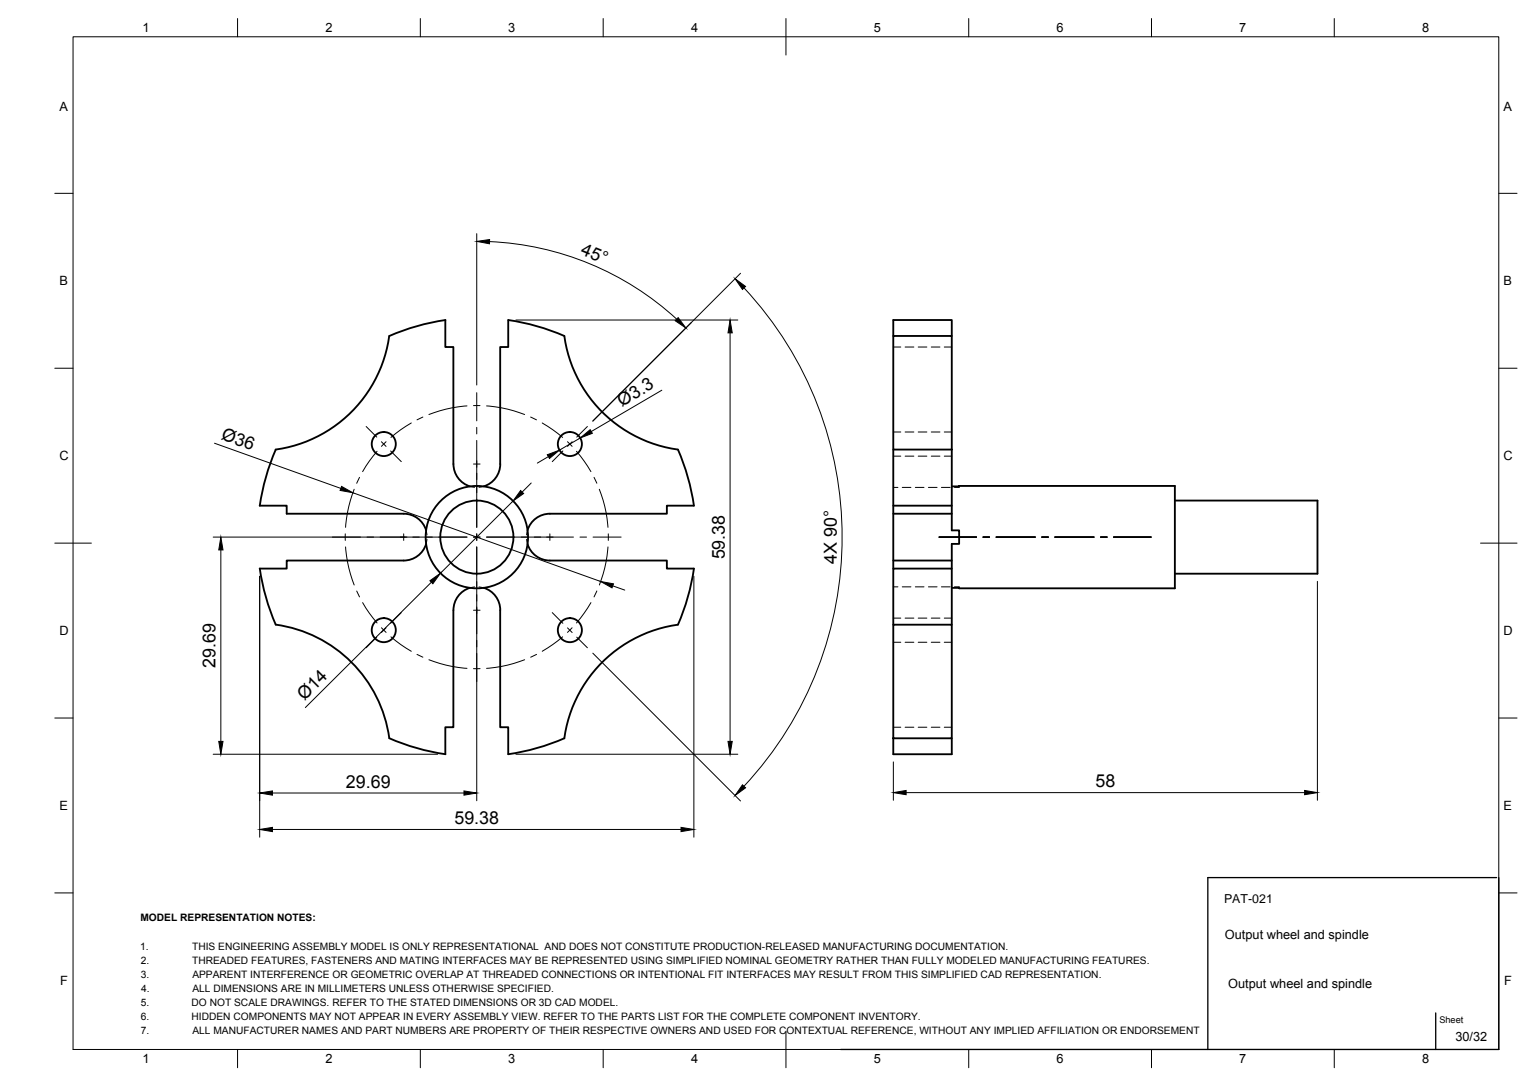
ISO-10303-21;
HEADER;
/* Generated by software containing ST-Developer
 * from STEP Tools, Inc. (www.steptools.com) 
 */

FILE_DESCRIPTION(
/* description */ ('Chain-less indexing wheel (Geneva) drive'),
/* implementation_level */ '2;1');

FILE_NAME(
/* name */ 'Output wheel and spindle.step',
/* time_stamp */ '2026-10-28T03:25:22-07:00',
/* author */ (''),
/* organization */ (''),
/* preprocessor_version */ 'ST-DEVELOPER v20.2',
/* originating_system */ 'Autodesk Translation Framework v15.17.0.0',
/* authorisation */ '');

FILE_SCHEMA (('AUTOMOTIVE_DESIGN { 1 0 10303 214 3 1 1 }'));
ENDSEC;

DATA;
#10=MECHANICAL_DESIGN_GEOMETRIC_PRESENTATION_REPRESENTATION('',(#332),#10957);
#274=SHAPE_REPRESENTATION_RELATIONSHIP('SRR','None',#11090,#299);
#299=ADVANCED_BREP_SHAPE_REPRESENTATION('',(#363),#10953);
#332=STYLED_ITEM('',(#11280),#363);
#363=MANIFOLD_SOLID_BREP('Body1',#5730);
#456=FACE_BOUND('',#1337,.T.);
#457=FACE_BOUND('',#1338,.T.);
#458=FACE_BOUND('',#1339,.T.);
#459=FACE_BOUND('',#1340,.T.);
#460=FACE_BOUND('',#1349,.T.);
#461=FACE_BOUND('',#1351,.T.);
#462=FACE_BOUND('',#1363,.T.);
#463=FACE_BOUND('',#1374,.T.);
#464=FACE_BOUND('',#1388,.T.);
#600=PLANE('',#6604);
#601=PLANE('',#6618);
#602=PLANE('',#6619);
#603=PLANE('',#6620);
#604=PLANE('',#6621);
#605=PLANE('',#6622);
#606=PLANE('',#6623);
#607=PLANE('',#6628);
#608=PLANE('',#6632);
#609=PLANE('',#6644);
#610=PLANE('',#6646);
#611=PLANE('',#6647);
#612=PLANE('',#6648);
#613=PLANE('',#6649);
#614=PLANE('',#6650);
#615=PLANE('',#6651);
#616=PLANE('',#6655);
#617=PLANE('',#6658);
#618=PLANE('',#6660);
#619=PLANE('',#6661);
#620=PLANE('',#6662);
#621=PLANE('',#6663);
#622=PLANE('',#6664);
#623=PLANE('',#6665);
#624=PLANE('',#6669);
#625=PLANE('',#6672);
#626=PLANE('',#6674);
#627=PLANE('',#6675);
#628=PLANE('',#6676);
#629=PLANE('',#6677);
#630=PLANE('',#6678);
#631=PLANE('',#6681);
#632=PLANE('',#6682);
#633=PLANE('',#6683);
#634=PLANE('',#6687);
#903=FACE_OUTER_BOUND('',#1325,.T.);
#904=FACE_OUTER_BOUND('',#1326,.T.);
#905=FACE_OUTER_BOUND('',#1327,.T.);
#906=FACE_OUTER_BOUND('',#1328,.T.);
#907=FACE_OUTER_BOUND('',#1329,.T.);
#908=FACE_OUTER_BOUND('',#1330,.T.);
#909=FACE_OUTER_BOUND('',#1331,.T.);
#910=FACE_OUTER_BOUND('',#1332,.T.);
#911=FACE_OUTER_BOUND('',#1333,.T.);
#912=FACE_OUTER_BOUND('',#1334,.T.);
#913=FACE_OUTER_BOUND('',#1335,.T.);
#914=FACE_OUTER_BOUND('',#1336,.T.);
#915=FACE_OUTER_BOUND('',#1341,.T.);
#916=FACE_OUTER_BOUND('',#1342,.T.);
#917=FACE_OUTER_BOUND('',#1343,.T.);
#918=FACE_OUTER_BOUND('',#1344,.T.);
#919=FACE_OUTER_BOUND('',#1345,.T.);
#920=FACE_OUTER_BOUND('',#1346,.T.);
#921=FACE_OUTER_BOUND('',#1347,.T.);
#922=FACE_OUTER_BOUND('',#1348,.T.);
#923=FACE_OUTER_BOUND('',#1350,.T.);
#924=FACE_OUTER_BOUND('',#1352,.T.);
#925=FACE_OUTER_BOUND('',#1353,.T.);
#926=FACE_OUTER_BOUND('',#1354,.T.);
#927=FACE_OUTER_BOUND('',#1355,.T.);
#928=FACE_OUTER_BOUND('',#1356,.T.);
#929=FACE_OUTER_BOUND('',#1357,.T.);
#930=FACE_OUTER_BOUND('',#1358,.T.);
#931=FACE_OUTER_BOUND('',#1359,.T.);
#932=FACE_OUTER_BOUND('',#1360,.T.);
#933=FACE_OUTER_BOUND('',#1361,.T.);
#934=FACE_OUTER_BOUND('',#1362,.T.);
#935=FACE_OUTER_BOUND('',#1364,.T.);
#936=FACE_OUTER_BOUND('',#1365,.T.);
#937=FACE_OUTER_BOUND('',#1366,.T.);
#938=FACE_OUTER_BOUND('',#1367,.T.);
#939=FACE_OUTER_BOUND('',#1368,.T.);
#940=FACE_OUTER_BOUND('',#1369,.T.);
#941=FACE_OUTER_BOUND('',#1370,.T.);
#942=FACE_OUTER_BOUND('',#1371,.T.);
#943=FACE_OUTER_BOUND('',#1372,.T.);
#944=FACE_OUTER_BOUND('',#1373,.T.);
#945=FACE_OUTER_BOUND('',#1375,.T.);
#946=FACE_OUTER_BOUND('',#1376,.T.);
#947=FACE_OUTER_BOUND('',#1377,.T.);
#948=FACE_OUTER_BOUND('',#1378,.T.);
#949=FACE_OUTER_BOUND('',#1379,.T.);
#950=FACE_OUTER_BOUND('',#1380,.T.);
#951=FACE_OUTER_BOUND('',#1381,.T.);
#952=FACE_OUTER_BOUND('',#1382,.T.);
#953=FACE_OUTER_BOUND('',#1383,.T.);
#954=FACE_OUTER_BOUND('',#1384,.T.);
#955=FACE_OUTER_BOUND('',#1385,.T.);
#956=FACE_OUTER_BOUND('',#1386,.T.);
#957=FACE_OUTER_BOUND('',#1387,.T.);
#958=FACE_OUTER_BOUND('',#1389,.T.);
#959=FACE_OUTER_BOUND('',#1390,.T.);
#1325=EDGE_LOOP('',(#4803,#4804,#4805,#4806));
#1326=EDGE_LOOP('',(#4807,#4808,#4809,#4810));
#1327=EDGE_LOOP('',(#4811,#4812,#4813,#4814));
#1328=EDGE_LOOP('',(#4815,#4816,#4817,#4818));
#1329=EDGE_LOOP('',(#4819,#4820,#4821,#4822));
#1330=EDGE_LOOP('',(#4823,#4824,#4825,#4826));
#1331=EDGE_LOOP('',(#4827,#4828,#4829,#4830));
#1332=EDGE_LOOP('',(#4831,#4832,#4833,#4834));
#1333=EDGE_LOOP('',(#4835,#4836,#4837,#4838));
#1334=EDGE_LOOP('',(#4839,#4840,#4841,#4842));
#1335=EDGE_LOOP('',(#4843,#4844,#4845,#4846));
#1336=EDGE_LOOP('',(#4847,#4848,#4849,#4850,#4851,#4852,#4853,#4854,#4855,
#4856,#4857,#4858,#4859,#4860,#4861,#4862,#4863,#4864,#4865,#4866,#4867,
#4868,#4869,#4870,#4871,#4872,#4873,#4874,#4875,#4876,#4877,#4878,#4879,
#4880,#4881,#4882,#4883,#4884,#4885,#4886));
#1337=EDGE_LOOP('',(#4887));
#1338=EDGE_LOOP('',(#4888));
#1339=EDGE_LOOP('',(#4889));
#1340=EDGE_LOOP('',(#4890));
#1341=EDGE_LOOP('',(#4891,#4892,#4893,#4894));
#1342=EDGE_LOOP('',(#4895,#4896,#4897,#4898));
#1343=EDGE_LOOP('',(#4899,#4900,#4901,#4902));
#1344=EDGE_LOOP('',(#4903,#4904,#4905,#4906));
#1345=EDGE_LOOP('',(#4907,#4908,#4909,#4910));
#1346=EDGE_LOOP('',(#4911,#4912,#4913,#4914));
#1347=EDGE_LOOP('',(#4915,#4916,#4917,#4918));
#1348=EDGE_LOOP('',(#4919,#4920,#4921,#4922,#4923,#4924,#4925,#4926,#4927,
#4928,#4929,#4930));
#1349=EDGE_LOOP('',(#4931));
#1350=EDGE_LOOP('',(#4932,#4933,#4934,#4935,#4936,#4937,#4938,#4939,#4940,
#4941,#4942,#4943));
#1351=EDGE_LOOP('',(#4944));
#1352=EDGE_LOOP('',(#4945,#4946));
#1353=EDGE_LOOP('',(#4947,#4948,#4949,#4950,#4951,#4952,#4953,#4954));
#1354=EDGE_LOOP('',(#4955,#4956,#4957,#4958,#4959,#4960,#4961,#4962,#4963,
#4964,#4965,#4966,#4967,#4968,#4969,#4970,#4971,#4972,#4973,#4974));
#1355=EDGE_LOOP('',(#4975,#4976,#4977,#4978));
#1356=EDGE_LOOP('',(#4979,#4980,#4981,#4982));
#1357=EDGE_LOOP('',(#4983,#4984,#4985,#4986));
#1358=EDGE_LOOP('',(#4987,#4988,#4989,#4990));
#1359=EDGE_LOOP('',(#4991,#4992,#4993,#4994));
#1360=EDGE_LOOP('',(#4995,#4996,#4997,#4998));
#1361=EDGE_LOOP('',(#4999,#5000,#5001,#5002));
#1362=EDGE_LOOP('',(#5003,#5004,#5005,#5006,#5007,#5008,#5009,#5010,#5011,
#5012,#5013,#5014));
#1363=EDGE_LOOP('',(#5015));
#1364=EDGE_LOOP('',(#5016,#5017,#5018));
#1365=EDGE_LOOP('',(#5019,#5020,#5021,#5022,#5023,#5024,#5025,#5026));
#1366=EDGE_LOOP('',(#5027,#5028,#5029,#5030));
#1367=EDGE_LOOP('',(#5031,#5032,#5033,#5034));
#1368=EDGE_LOOP('',(#5035,#5036,#5037,#5038));
#1369=EDGE_LOOP('',(#5039,#5040,#5041,#5042));
#1370=EDGE_LOOP('',(#5043,#5044,#5045,#5046));
#1371=EDGE_LOOP('',(#5047,#5048,#5049,#5050));
#1372=EDGE_LOOP('',(#5051,#5052,#5053,#5054));
#1373=EDGE_LOOP('',(#5055,#5056,#5057,#5058,#5059,#5060,#5061,#5062,#5063,
#5064,#5065,#5066));
#1374=EDGE_LOOP('',(#5067));
#1375=EDGE_LOOP('',(#5068,#5069));
#1376=EDGE_LOOP('',(#5070,#5071,#5072,#5073,#5074,#5075,#5076,#5077));
#1377=EDGE_LOOP('',(#5078,#5079,#5080,#5081));
#1378=EDGE_LOOP('',(#5082,#5083,#5084,#5085));
#1379=EDGE_LOOP('',(#5086,#5087,#5088,#5089));
#1380=EDGE_LOOP('',(#5090,#5091,#5092,#5093));
#1381=EDGE_LOOP('',(#5094,#5095,#5096,#5097));
#1382=EDGE_LOOP('',(#5098,#5099,#5100,#5101));
#1383=EDGE_LOOP('',(#5102,#5103));
#1384=EDGE_LOOP('',(#5104,#5105,#5106,#5107,#5108,#5109,#5110,#5111));
#1385=EDGE_LOOP('',(#5112,#5113,#5114,#5115));
#1386=EDGE_LOOP('',(#5116,#5117,#5118,#5119));
#1387=EDGE_LOOP('',(#5120));
#1388=EDGE_LOOP('',(#5121));
#1389=EDGE_LOOP('',(#5122,#5123,#5124,#5125));
#1390=EDGE_LOOP('',(#5126));
#1663=LINE('',#10310,#2037);
#1664=LINE('',#10316,#2038);
#1665=LINE('',#10322,#2039);
#1666=LINE('',#10328,#2040);
#1667=LINE('',#10335,#2041);
#1668=LINE('',#10338,#2042);
#1669=LINE('',#10344,#2043);
#1670=LINE('',#10347,#2044);
#1671=LINE('',#10353,#2045);
#1672=LINE('',#10356,#2046);
#1673=LINE('',#10360,#2047);
#1674=LINE('',#10364,#2048);
#1675=LINE('',#10370,#2049);
#1676=LINE('',#10376,#2050);
#1677=LINE('',#10382,#2051);
#1678=LINE('',#10386,#2052);
#1679=LINE('',#10388,#2053);
#1680=LINE('',#10390,#2054);
#1681=LINE('',#10394,#2055);
#1682=LINE('',#10396,#2056);
#1683=LINE('',#10398,#2057);
#1684=LINE('',#10403,#2058);
#1685=LINE('',#10405,#2059);
#1686=LINE('',#10407,#2060);
#1687=LINE('',#10411,#2061);
#1688=LINE('',#10413,#2062);
#1689=LINE('',#10415,#2063);
#1690=LINE('',#10418,#2064);
#1691=LINE('',#10420,#2065);
#1692=LINE('',#10422,#2066);
#1693=LINE('',#10426,#2067);
#1694=LINE('',#10428,#2068);
#1695=LINE('',#10430,#2069);
#1696=LINE('',#10433,#2070);
#1697=LINE('',#10435,#2071);
#1698=LINE('',#10437,#2072);
#1699=LINE('',#10441,#2073);
#1700=LINE('',#10443,#2074);
#1701=LINE('',#10445,#2075);
#1702=LINE('',#10450,#2076);
#1703=LINE('',#10453,#2077);
#1704=LINE('',#10457,#2078);
#1705=LINE('',#10458,#2079);
#1706=LINE('',#10461,#2080);
#1707=LINE('',#10462,#2081);
#1708=LINE('',#10465,#2082);
#1709=LINE('',#10467,#2083);
#1710=LINE('',#10468,#2084);
#1711=LINE('',#10470,#2085);
#1712=LINE('',#10473,#2086);
#1713=LINE('',#10474,#2087);
#1714=LINE('',#10479,#2088);
#1715=LINE('',#10481,#2089);
#1716=LINE('',#10483,#2090);
#1717=LINE('',#10491,#2091);
#1718=LINE('',#10499,#2092);
#1719=LINE('',#10501,#2093);
#1720=LINE('',#10502,#2094);
#1721=LINE('',#10509,#2095);
#1722=LINE('',#10510,#2096);
#1723=LINE('',#10511,#2097);
#1724=LINE('',#10514,#2098);
#1725=LINE('',#10518,#2099);
#1726=LINE('',#10523,#2100);
#1727=LINE('',#10527,#2101);
#1728=LINE('',#10531,#2102);
#1729=LINE('',#10535,#2103);
#1730=LINE('',#10538,#2104);
#1731=LINE('',#10541,#2105);
#1732=LINE('',#10543,#2106);
#1733=LINE('',#10545,#2107);
#1734=LINE('',#10548,#2108);
#1735=LINE('',#10550,#2109);
#1736=LINE('',#10551,#2110);
#1737=LINE('',#10553,#2111);
#1738=LINE('',#10556,#2112);
#1739=LINE('',#10557,#2113);
#1740=LINE('',#10562,#2114);
#1741=LINE('',#10564,#2115);
#1742=LINE('',#10566,#2116);
#1743=LINE('',#10572,#2117);
#1744=LINE('',#10575,#2118);
#1745=LINE('',#10577,#2119);
#1746=LINE('',#10579,#2120);
#1747=LINE('',#10582,#2121);
#1748=LINE('',#10584,#2122);
#1749=LINE('',#10585,#2123);
#1750=LINE('',#10587,#2124);
#1751=LINE('',#10590,#2125);
#1752=LINE('',#10591,#2126);
#1753=LINE('',#10596,#2127);
#1754=LINE('',#10598,#2128);
#1755=LINE('',#10600,#2129);
#1756=LINE('',#10606,#2130);
#1757=LINE('',#10609,#2131);
#1758=LINE('',#10611,#2132);
#1759=LINE('',#10613,#2133);
#1760=LINE('',#10615,#2134);
#1761=LINE('',#10617,#2135);
#1762=LINE('',#10621,#2136);
#1763=LINE('',#10622,#2137);
#1764=LINE('',#10630,#2138);
#2037=VECTOR('',#8115,0.165);
#2038=VECTOR('',#8122,0.165);
#2039=VECTOR('',#8129,0.165);
#2040=VECTOR('',#8136,0.165);
#2041=VECTOR('',#8143,1.);
#2042=VECTOR('',#8146,1.);
#2043=VECTOR('',#8151,1.);
#2044=VECTOR('',#8154,1.);
#2045=VECTOR('',#8159,1.);
#2046=VECTOR('',#8162,1.);
#2047=VECTOR('',#8165,1.);
#2048=VECTOR('',#8168,1.);
#2049=VECTOR('',#8175,1.);
#2050=VECTOR('',#8182,1.);
#2051=VECTOR('',#8189,1.);
#2052=VECTOR('',#8194,1.);
#2053=VECTOR('',#8195,1.);
#2054=VECTOR('',#8196,1.);
#2055=VECTOR('',#8199,1.);
#2056=VECTOR('',#8200,1.);
#2057=VECTOR('',#8201,1.);
#2058=VECTOR('',#8206,1.);
#2059=VECTOR('',#8207,1.);
#2060=VECTOR('',#8208,1.);
#2061=VECTOR('',#8211,1.);
#2062=VECTOR('',#8212,1.);
#2063=VECTOR('',#8213,1.);
#2064=VECTOR('',#8216,1.);
#2065=VECTOR('',#8217,1.);
#2066=VECTOR('',#8218,1.);
#2067=VECTOR('',#8221,1.);
#2068=VECTOR('',#8222,1.);
#2069=VECTOR('',#8223,1.);
#2070=VECTOR('',#8226,1.);
#2071=VECTOR('',#8227,1.);
#2072=VECTOR('',#8228,1.);
#2073=VECTOR('',#8231,1.);
#2074=VECTOR('',#8232,1.);
#2075=VECTOR('',#8233,1.);
#2076=VECTOR('',#8240,1.);
#2077=VECTOR('',#8243,1.);
#2078=VECTOR('',#8248,1.);
#2079=VECTOR('',#8249,1.);
#2080=VECTOR('',#8252,1.);
#2081=VECTOR('',#8253,1.);
#2082=VECTOR('',#8256,1.);
#2083=VECTOR('',#8257,1.);
#2084=VECTOR('',#8258,1.);
#2085=VECTOR('',#8261,1.);
#2086=VECTOR('',#8264,1.);
#2087=VECTOR('',#8265,1.);
#2088=VECTOR('',#8270,1.);
#2089=VECTOR('',#8271,1.);
#2090=VECTOR('',#8272,1.);
#2091=VECTOR('',#8281,1.);
#2092=VECTOR('',#8288,1.);
#2093=VECTOR('',#8289,1.);
#2094=VECTOR('',#8290,1.);
#2095=VECTOR('',#8299,1.);
#2096=VECTOR('',#8300,1.);
#2097=VECTOR('',#8301,1.);
#2098=VECTOR('',#8304,1.);
#2099=VECTOR('',#8307,0.7);
#2100=VECTOR('',#8312,1.);
#2101=VECTOR('',#8315,1.);
#2102=VECTOR('',#8318,1.);
#2103=VECTOR('',#8321,1.);
#2104=VECTOR('',#8324,1.);
#2105=VECTOR('',#8329,1.);
#2106=VECTOR('',#8332,1.);
#2107=VECTOR('',#8335,1.);
#2108=VECTOR('',#8338,1.);
#2109=VECTOR('',#8339,1.);
#2110=VECTOR('',#8340,1.);
#2111=VECTOR('',#8343,1.);
#2112=VECTOR('',#8346,1.);
#2113=VECTOR('',#8347,1.);
#2114=VECTOR('',#8352,1.);
#2115=VECTOR('',#8353,1.);
#2116=VECTOR('',#8354,1.);
#2117=VECTOR('',#8365,1.);
#2118=VECTOR('',#8370,1.);
#2119=VECTOR('',#8373,1.);
#2120=VECTOR('',#8376,1.);
#2121=VECTOR('',#8379,1.);
#2122=VECTOR('',#8380,1.);
#2123=VECTOR('',#8381,1.);
#2124=VECTOR('',#8384,1.);
#2125=VECTOR('',#8387,1.);
#2126=VECTOR('',#8388,1.);
#2127=VECTOR('',#8393,1.);
#2128=VECTOR('',#8394,1.);
#2129=VECTOR('',#8395,1.);
#2130=VECTOR('',#8406,1.);
#2131=VECTOR('',#8411,1.);
#2132=VECTOR('',#8414,1.);
#2133=VECTOR('',#8417,1.);
#2134=VECTOR('',#8420,1.);
#2135=VECTOR('',#8423,1.);
#2136=VECTOR('',#8430,1.);
#2137=VECTOR('',#8431,1.);
#2138=VECTOR('',#8442,0.5);
#2429=CIRCLE('',#6572,0.165);
#2430=CIRCLE('',#6573,0.165);
#2431=CIRCLE('',#6575,0.165);
#2432=CIRCLE('',#6576,0.165);
#2433=CIRCLE('',#6578,0.165);
#2434=CIRCLE('',#6579,0.165);
#2435=CIRCLE('',#6581,0.165);
#2436=CIRCLE('',#6582,0.165);
#2437=CIRCLE('',#6584,1.82);
#2438=CIRCLE('',#6585,1.82);
#2439=CIRCLE('',#6587,1.82);
#2440=CIRCLE('',#6588,1.82);
#2441=CIRCLE('',#6590,1.82);
#2442=CIRCLE('',#6591,1.82);
#2443=CIRCLE('',#6593,1.82);
#2444=CIRCLE('',#6594,1.82);
#2445=CIRCLE('',#6596,3.);
#2446=CIRCLE('',#6597,3.);
#2447=CIRCLE('',#6599,3.);
#2448=CIRCLE('',#6600,3.);
#2449=CIRCLE('',#6602,3.);
#2450=CIRCLE('',#6603,3.);
#2451=CIRCLE('',#6605,0.32);
#2452=CIRCLE('',#6606,3.);
#2453=CIRCLE('',#6607,3.);
#2454=CIRCLE('',#6608,0.32);
#2455=CIRCLE('',#6609,3.);
#2456=CIRCLE('',#6610,0.32);
#2457=CIRCLE('',#6611,3.);
#2458=CIRCLE('',#6612,0.32);
#2459=CIRCLE('',#6613,3.);
#2460=CIRCLE('',#6615,3.);
#2461=CIRCLE('',#6617,3.);
#2462=CIRCLE('',#6624,3.);
#2463=CIRCLE('',#6625,0.32);
#2464=CIRCLE('',#6626,0.7);
#2465=CIRCLE('',#6627,0.32);
#2466=CIRCLE('',#6629,0.32);
#2467=CIRCLE('',#6630,0.7);
#2468=CIRCLE('',#6631,0.32);
#2469=CIRCLE('',#6633,0.7);
#2470=CIRCLE('',#6634,0.32);
#2471=CIRCLE('',#6637,0.7);
#2472=CIRCLE('',#6638,0.7);
#2473=CIRCLE('',#6639,0.7);
#2474=CIRCLE('',#6640,0.7);
#2475=CIRCLE('',#6641,0.7);
#2476=CIRCLE('',#6642,0.7);
#2477=CIRCLE('',#6643,0.7);
#2478=CIRCLE('',#6652,3.);
#2479=CIRCLE('',#6653,0.32);
#2480=CIRCLE('',#6654,0.32);
#2481=CIRCLE('',#6656,0.32);
#2482=CIRCLE('',#6666,3.);
#2483=CIRCLE('',#6667,0.32);
#2484=CIRCLE('',#6668,0.32);
#2485=CIRCLE('',#6670,0.32);
#2486=CIRCLE('',#6679,0.32);
#2487=CIRCLE('',#6684,0.5);
#2488=CIRCLE('',#6686,0.5);
#2853=VERTEX_POINT('',#10307);
#2854=VERTEX_POINT('',#10309);
#2855=VERTEX_POINT('',#10313);
#2856=VERTEX_POINT('',#10315);
#2857=VERTEX_POINT('',#10319);
#2858=VERTEX_POINT('',#10321);
#2859=VERTEX_POINT('',#10325);
#2860=VERTEX_POINT('',#10327);
#2861=VERTEX_POINT('',#10331);
#2862=VERTEX_POINT('',#10332);
#2863=VERTEX_POINT('',#10334);
#2864=VERTEX_POINT('',#10336);
#2865=VERTEX_POINT('',#10340);
#2866=VERTEX_POINT('',#10341);
#2867=VERTEX_POINT('',#10343);
#2868=VERTEX_POINT('',#10345);
#2869=VERTEX_POINT('',#10349);
#2870=VERTEX_POINT('',#10350);
#2871=VERTEX_POINT('',#10352);
#2872=VERTEX_POINT('',#10354);
#2873=VERTEX_POINT('',#10358);
#2874=VERTEX_POINT('',#10359);
#2875=VERTEX_POINT('',#10361);
#2876=VERTEX_POINT('',#10363);
#2877=VERTEX_POINT('',#10367);
#2878=VERTEX_POINT('',#10369);
#2879=VERTEX_POINT('',#10373);
#2880=VERTEX_POINT('',#10375);
#2881=VERTEX_POINT('',#10379);
#2882=VERTEX_POINT('',#10381);
#2883=VERTEX_POINT('',#10385);
#2884=VERTEX_POINT('',#10387);
#2885=VERTEX_POINT('',#10389);
#2886=VERTEX_POINT('',#10391);
#2887=VERTEX_POINT('',#10393);
#2888=VERTEX_POINT('',#10395);
#2889=VERTEX_POINT('',#10397);
#2890=VERTEX_POINT('',#10400);
#2891=VERTEX_POINT('',#10402);
#2892=VERTEX_POINT('',#10404);
#2893=VERTEX_POINT('',#10406);
#2894=VERTEX_POINT('',#10408);
#2895=VERTEX_POINT('',#10410);
#2896=VERTEX_POINT('',#10412);
#2897=VERTEX_POINT('',#10414);
#2898=VERTEX_POINT('',#10417);
#2899=VERTEX_POINT('',#10419);
#2900=VERTEX_POINT('',#10421);
#2901=VERTEX_POINT('',#10423);
#2902=VERTEX_POINT('',#10425);
#2903=VERTEX_POINT('',#10427);
#2904=VERTEX_POINT('',#10429);
#2905=VERTEX_POINT('',#10432);
#2906=VERTEX_POINT('',#10434);
#2907=VERTEX_POINT('',#10436);
#2908=VERTEX_POINT('',#10438);
#2909=VERTEX_POINT('',#10440);
#2910=VERTEX_POINT('',#10442);
#2911=VERTEX_POINT('',#10444);
#2912=VERTEX_POINT('',#10448);
#2913=VERTEX_POINT('',#10452);
#2914=VERTEX_POINT('',#10456);
#2915=VERTEX_POINT('',#10460);
#2916=VERTEX_POINT('',#10464);
#2917=VERTEX_POINT('',#10466);
#2918=VERTEX_POINT('',#10472);
#2919=VERTEX_POINT('',#10476);
#2920=VERTEX_POINT('',#10478);
#2921=VERTEX_POINT('',#10480);
#2922=VERTEX_POINT('',#10482);
#2923=VERTEX_POINT('',#10484);
#2924=VERTEX_POINT('',#10486);
#2925=VERTEX_POINT('',#10490);
#2926=VERTEX_POINT('',#10492);
#2927=VERTEX_POINT('',#10494);
#2928=VERTEX_POINT('',#10496);
#2929=VERTEX_POINT('',#10498);
#2930=VERTEX_POINT('',#10500);
#2931=VERTEX_POINT('',#10504);
#2932=VERTEX_POINT('',#10505);
#2933=VERTEX_POINT('',#10513);
#2934=VERTEX_POINT('',#10515);
#2935=VERTEX_POINT('',#10517);
#2936=VERTEX_POINT('',#10520);
#2937=VERTEX_POINT('',#10522);
#2938=VERTEX_POINT('',#10524);
#2939=VERTEX_POINT('',#10526);
#2940=VERTEX_POINT('',#10528);
#2941=VERTEX_POINT('',#10530);
#2942=VERTEX_POINT('',#10532);
#2943=VERTEX_POINT('',#10534);
#2944=VERTEX_POINT('',#10536);
#2945=VERTEX_POINT('',#10547);
#2946=VERTEX_POINT('',#10549);
#2947=VERTEX_POINT('',#10555);
#2948=VERTEX_POINT('',#10559);
#2949=VERTEX_POINT('',#10561);
#2950=VERTEX_POINT('',#10563);
#2951=VERTEX_POINT('',#10565);
#2952=VERTEX_POINT('',#10581);
#2953=VERTEX_POINT('',#10583);
#2954=VERTEX_POINT('',#10589);
#2955=VERTEX_POINT('',#10593);
#2956=VERTEX_POINT('',#10595);
#2957=VERTEX_POINT('',#10597);
#2958=VERTEX_POINT('',#10599);
#2959=VERTEX_POINT('',#10626);
#2960=VERTEX_POINT('',#10629);
#3527=EDGE_CURVE('',#2853,#2853,#2429,.T.);
#3528=EDGE_CURVE('',#2853,#2854,#1663,.T.);
#3529=EDGE_CURVE('',#2854,#2854,#2430,.T.);
#3530=EDGE_CURVE('',#2855,#2855,#2431,.T.);
#3531=EDGE_CURVE('',#2855,#2856,#1664,.T.);
#3532=EDGE_CURVE('',#2856,#2856,#2432,.T.);
#3533=EDGE_CURVE('',#2857,#2857,#2433,.T.);
#3534=EDGE_CURVE('',#2857,#2858,#1665,.T.);
#3535=EDGE_CURVE('',#2858,#2858,#2434,.T.);
#3536=EDGE_CURVE('',#2859,#2859,#2435,.T.);
#3537=EDGE_CURVE('',#2859,#2860,#1666,.T.);
#3538=EDGE_CURVE('',#2860,#2860,#2436,.T.);
#3539=EDGE_CURVE('',#2861,#2862,#2437,.T.);
#3540=EDGE_CURVE('',#2863,#2861,#1667,.T.);
#3541=EDGE_CURVE('',#2864,#2863,#2438,.T.);
#3542=EDGE_CURVE('',#2862,#2864,#1668,.T.);
#3543=EDGE_CURVE('',#2865,#2866,#2439,.T.);
#3544=EDGE_CURVE('',#2867,#2865,#1669,.T.);
#3545=EDGE_CURVE('',#2868,#2867,#2440,.T.);
#3546=EDGE_CURVE('',#2866,#2868,#1670,.T.);
#3547=EDGE_CURVE('',#2869,#2870,#2441,.T.);
#3548=EDGE_CURVE('',#2871,#2869,#1671,.T.);
#3549=EDGE_CURVE('',#2872,#2871,#2442,.T.);
#3550=EDGE_CURVE('',#2870,#2872,#1672,.T.);
#3551=EDGE_CURVE('',#2873,#2874,#1673,.T.);
#3552=EDGE_CURVE('',#2875,#2873,#2443,.T.);
#3553=EDGE_CURVE('',#2876,#2875,#1674,.T.);
#3554=EDGE_CURVE('',#2874,#2876,#2444,.T.);
#3555=EDGE_CURVE('',#2861,#2877,#2445,.T.);
#3556=EDGE_CURVE('',#2877,#2878,#1675,.T.);
#3557=EDGE_CURVE('',#2863,#2878,#2446,.T.);
#3558=EDGE_CURVE('',#2865,#2879,#2447,.T.);
#3559=EDGE_CURVE('',#2879,#2880,#1676,.T.);
#3560=EDGE_CURVE('',#2867,#2880,#2448,.T.);
#3561=EDGE_CURVE('',#2869,#2881,#2449,.T.);
#3562=EDGE_CURVE('',#2881,#2882,#1677,.T.);
#3563=EDGE_CURVE('',#2871,#2882,#2450,.T.);
#3564=EDGE_CURVE('',#2878,#2883,#1678,.T.);
#3565=EDGE_CURVE('',#2883,#2884,#1679,.T.);
#3566=EDGE_CURVE('',#2884,#2885,#1680,.T.);
#3567=EDGE_CURVE('',#2885,#2886,#2451,.T.);
#3568=EDGE_CURVE('',#2886,#2887,#1681,.T.);
#3569=EDGE_CURVE('',#2887,#2888,#1682,.T.);
#3570=EDGE_CURVE('',#2888,#2889,#1683,.T.);
#3571=EDGE_CURVE('',#2889,#2875,#2452,.T.);
#3572=EDGE_CURVE('',#2873,#2890,#2453,.T.);
#3573=EDGE_CURVE('',#2890,#2891,#1684,.T.);
#3574=EDGE_CURVE('',#2891,#2892,#1685,.T.);
#3575=EDGE_CURVE('',#2892,#2893,#1686,.T.);
#3576=EDGE_CURVE('',#2893,#2894,#2454,.T.);
#3577=EDGE_CURVE('',#2894,#2895,#1687,.T.);
#3578=EDGE_CURVE('',#2895,#2896,#1688,.T.);
#3579=EDGE_CURVE('',#2896,#2897,#1689,.T.);
#3580=EDGE_CURVE('',#2897,#2872,#2455,.T.);
#3581=EDGE_CURVE('',#2882,#2898,#1690,.T.);
#3582=EDGE_CURVE('',#2898,#2899,#1691,.T.);
#3583=EDGE_CURVE('',#2899,#2900,#1692,.T.);
#3584=EDGE_CURVE('',#2900,#2901,#2456,.T.);
#3585=EDGE_CURVE('',#2901,#2902,#1693,.T.);
#3586=EDGE_CURVE('',#2902,#2903,#1694,.T.);
#3587=EDGE_CURVE('',#2903,#2904,#1695,.T.);
#3588=EDGE_CURVE('',#2904,#2868,#2457,.T.);
#3589=EDGE_CURVE('',#2880,#2905,#1696,.T.);
#3590=EDGE_CURVE('',#2905,#2906,#1697,.T.);
#3591=EDGE_CURVE('',#2906,#2907,#1698,.T.);
#3592=EDGE_CURVE('',#2907,#2908,#2458,.T.);
#3593=EDGE_CURVE('',#2908,#2909,#1699,.T.);
#3594=EDGE_CURVE('',#2909,#2910,#1700,.T.);
#3595=EDGE_CURVE('',#2910,#2911,#1701,.T.);
#3596=EDGE_CURVE('',#2911,#2864,#2459,.T.);
#3597=EDGE_CURVE('',#2874,#2912,#2460,.T.);
#3598=EDGE_CURVE('',#2912,#2890,#1702,.T.);
#3599=EDGE_CURVE('',#2889,#2913,#1703,.T.);
#3600=EDGE_CURVE('',#2913,#2876,#2461,.T.);
#3601=EDGE_CURVE('',#2914,#2888,#1704,.T.);
#3602=EDGE_CURVE('',#2913,#2914,#1705,.T.);
#3603=EDGE_CURVE('',#2915,#2887,#1706,.T.);
#3604=EDGE_CURVE('',#2914,#2915,#1707,.T.);
#3605=EDGE_CURVE('',#2916,#2883,#1708,.T.);
#3606=EDGE_CURVE('',#2917,#2916,#1709,.T.);
#3607=EDGE_CURVE('',#2884,#2917,#1710,.T.);
#3608=EDGE_CURVE('',#2916,#2877,#1711,.T.);
#3609=EDGE_CURVE('',#2918,#2917,#1712,.T.);
#3610=EDGE_CURVE('',#2918,#2885,#1713,.T.);
#3611=EDGE_CURVE('',#2919,#2862,#2462,.T.);
#3612=EDGE_CURVE('',#2919,#2920,#1714,.T.);
#3613=EDGE_CURVE('',#2920,#2921,#1715,.T.);
#3614=EDGE_CURVE('',#2921,#2922,#1716,.T.);
#3615=EDGE_CURVE('',#2922,#2923,#2463,.T.);
#3616=EDGE_CURVE('',#2923,#2924,#2464,.T.);
#3617=EDGE_CURVE('',#2924,#2918,#2465,.T.);
#3618=EDGE_CURVE('',#2915,#2925,#1717,.T.);
#3619=EDGE_CURVE('',#2925,#2926,#2466,.T.);
#3620=EDGE_CURVE('',#2926,#2927,#2467,.T.);
#3621=EDGE_CURVE('',#2927,#2928,#2468,.T.);
#3622=EDGE_CURVE('',#2928,#2929,#1718,.T.);
#3623=EDGE_CURVE('',#2929,#2930,#1719,.T.);
#3624=EDGE_CURVE('',#2930,#2912,#1720,.T.);
#3625=EDGE_CURVE('',#2931,#2932,#2469,.T.);
#3626=EDGE_CURVE('',#2931,#2932,#2470,.T.);
#3627=EDGE_CURVE('',#2926,#2931,#1721,.T.);
#3628=EDGE_CURVE('',#2925,#2886,#1722,.T.);
#3629=EDGE_CURVE('',#2932,#2924,#1723,.T.);
#3630=EDGE_CURVE('',#2923,#2933,#1724,.T.);
#3631=EDGE_CURVE('',#2933,#2934,#2471,.T.);
#3632=EDGE_CURVE('',#2934,#2935,#1725,.T.);
#3633=EDGE_CURVE('',#2935,#2935,#2472,.T.);
#3634=EDGE_CURVE('',#2934,#2936,#2473,.T.);
#3635=EDGE_CURVE('',#2936,#2937,#1726,.T.);
#3636=EDGE_CURVE('',#2938,#2937,#2474,.T.);
#3637=EDGE_CURVE('',#2938,#2939,#1727,.T.);
#3638=EDGE_CURVE('',#2939,#2940,#2475,.T.);
#3639=EDGE_CURVE('',#2940,#2941,#1728,.T.);
#3640=EDGE_CURVE('',#2942,#2941,#2476,.T.);
#3641=EDGE_CURVE('',#2942,#2943,#1729,.T.);
#3642=EDGE_CURVE('',#2943,#2944,#2477,.T.);
#3643=EDGE_CURVE('',#2944,#2927,#1730,.T.);
#3644=EDGE_CURVE('',#2911,#2919,#1731,.T.);
#3645=EDGE_CURVE('',#2920,#2910,#1732,.T.);
#3646=EDGE_CURVE('',#2921,#2909,#1733,.T.);
#3647=EDGE_CURVE('',#2945,#2905,#1734,.T.);
#3648=EDGE_CURVE('',#2946,#2945,#1735,.T.);
#3649=EDGE_CURVE('',#2906,#2946,#1736,.T.);
#3650=EDGE_CURVE('',#2945,#2879,#1737,.T.);
#3651=EDGE_CURVE('',#2947,#2946,#1738,.T.);
#3652=EDGE_CURVE('',#2947,#2907,#1739,.T.);
#3653=EDGE_CURVE('',#2948,#2866,#2478,.T.);
#3654=EDGE_CURVE('',#2948,#2949,#1740,.T.);
#3655=EDGE_CURVE('',#2949,#2950,#1741,.T.);
#3656=EDGE_CURVE('',#2950,#2951,#1742,.T.);
#3657=EDGE_CURVE('',#2951,#2938,#2479,.T.);
#3658=EDGE_CURVE('',#2937,#2947,#2480,.T.);
#3659=EDGE_CURVE('',#2933,#2936,#2481,.T.);
#3660=EDGE_CURVE('',#2922,#2908,#1743,.T.);
#3661=EDGE_CURVE('',#2904,#2948,#1744,.T.);
#3662=EDGE_CURVE('',#2949,#2903,#1745,.T.);
#3663=EDGE_CURVE('',#2950,#2902,#1746,.T.);
#3664=EDGE_CURVE('',#2952,#2898,#1747,.T.);
#3665=EDGE_CURVE('',#2953,#2952,#1748,.T.);
#3666=EDGE_CURVE('',#2899,#2953,#1749,.T.);
#3667=EDGE_CURVE('',#2952,#2881,#1750,.T.);
#3668=EDGE_CURVE('',#2954,#2953,#1751,.T.);
#3669=EDGE_CURVE('',#2954,#2900,#1752,.T.);
#3670=EDGE_CURVE('',#2955,#2870,#2482,.T.);
#3671=EDGE_CURVE('',#2955,#2956,#1753,.T.);
#3672=EDGE_CURVE('',#2956,#2957,#1754,.T.);
#3673=EDGE_CURVE('',#2957,#2958,#1755,.T.);
#3674=EDGE_CURVE('',#2958,#2942,#2483,.T.);
#3675=EDGE_CURVE('',#2941,#2954,#2484,.T.);
#3676=EDGE_CURVE('',#2939,#2940,#2485,.T.);
#3677=EDGE_CURVE('',#2951,#2901,#1756,.T.);
#3678=EDGE_CURVE('',#2897,#2955,#1757,.T.);
#3679=EDGE_CURVE('',#2956,#2896,#1758,.T.);
#3680=EDGE_CURVE('',#2930,#2891,#1759,.T.);
#3681=EDGE_CURVE('',#2892,#2929,#1760,.T.);
#3682=EDGE_CURVE('',#2957,#2895,#1761,.T.);
#3683=EDGE_CURVE('',#2943,#2944,#2486,.T.);
#3684=EDGE_CURVE('',#2958,#2894,#1762,.T.);
#3685=EDGE_CURVE('',#2928,#2893,#1763,.T.);
#3686=EDGE_CURVE('',#2959,#2959,#2487,.T.);
#3687=EDGE_CURVE('',#2959,#2960,#1764,.T.);
#3688=EDGE_CURVE('',#2960,#2960,#2488,.T.);
#4803=ORIENTED_EDGE('',*,*,#3527,.F.);
#4804=ORIENTED_EDGE('',*,*,#3528,.T.);
#4805=ORIENTED_EDGE('',*,*,#3529,.F.);
#4806=ORIENTED_EDGE('',*,*,#3528,.F.);
#4807=ORIENTED_EDGE('',*,*,#3530,.F.);
#4808=ORIENTED_EDGE('',*,*,#3531,.T.);
#4809=ORIENTED_EDGE('',*,*,#3532,.F.);
#4810=ORIENTED_EDGE('',*,*,#3531,.F.);
#4811=ORIENTED_EDGE('',*,*,#3533,.F.);
#4812=ORIENTED_EDGE('',*,*,#3534,.T.);
#4813=ORIENTED_EDGE('',*,*,#3535,.F.);
#4814=ORIENTED_EDGE('',*,*,#3534,.F.);
#4815=ORIENTED_EDGE('',*,*,#3536,.F.);
#4816=ORIENTED_EDGE('',*,*,#3537,.T.);
#4817=ORIENTED_EDGE('',*,*,#3538,.F.);
#4818=ORIENTED_EDGE('',*,*,#3537,.F.);
#4819=ORIENTED_EDGE('',*,*,#3539,.F.);
#4820=ORIENTED_EDGE('',*,*,#3540,.F.);
#4821=ORIENTED_EDGE('',*,*,#3541,.F.);
#4822=ORIENTED_EDGE('',*,*,#3542,.F.);
#4823=ORIENTED_EDGE('',*,*,#3543,.F.);
#4824=ORIENTED_EDGE('',*,*,#3544,.F.);
#4825=ORIENTED_EDGE('',*,*,#3545,.F.);
#4826=ORIENTED_EDGE('',*,*,#3546,.F.);
#4827=ORIENTED_EDGE('',*,*,#3547,.F.);
#4828=ORIENTED_EDGE('',*,*,#3548,.F.);
#4829=ORIENTED_EDGE('',*,*,#3549,.F.);
#4830=ORIENTED_EDGE('',*,*,#3550,.F.);
#4831=ORIENTED_EDGE('',*,*,#3551,.F.);
#4832=ORIENTED_EDGE('',*,*,#3552,.F.);
#4833=ORIENTED_EDGE('',*,*,#3553,.F.);
#4834=ORIENTED_EDGE('',*,*,#3554,.F.);
#4835=ORIENTED_EDGE('',*,*,#3540,.T.);
#4836=ORIENTED_EDGE('',*,*,#3555,.T.);
#4837=ORIENTED_EDGE('',*,*,#3556,.T.);
#4838=ORIENTED_EDGE('',*,*,#3557,.F.);
#4839=ORIENTED_EDGE('',*,*,#3544,.T.);
#4840=ORIENTED_EDGE('',*,*,#3558,.T.);
#4841=ORIENTED_EDGE('',*,*,#3559,.T.);
#4842=ORIENTED_EDGE('',*,*,#3560,.F.);
#4843=ORIENTED_EDGE('',*,*,#3548,.T.);
#4844=ORIENTED_EDGE('',*,*,#3561,.T.);
#4845=ORIENTED_EDGE('',*,*,#3562,.T.);
#4846=ORIENTED_EDGE('',*,*,#3563,.F.);
#4847=ORIENTED_EDGE('',*,*,#3541,.T.);
#4848=ORIENTED_EDGE('',*,*,#3557,.T.);
#4849=ORIENTED_EDGE('',*,*,#3564,.T.);
#4850=ORIENTED_EDGE('',*,*,#3565,.T.);
#4851=ORIENTED_EDGE('',*,*,#3566,.T.);
#4852=ORIENTED_EDGE('',*,*,#3567,.T.);
#4853=ORIENTED_EDGE('',*,*,#3568,.T.);
#4854=ORIENTED_EDGE('',*,*,#3569,.T.);
#4855=ORIENTED_EDGE('',*,*,#3570,.T.);
#4856=ORIENTED_EDGE('',*,*,#3571,.T.);
#4857=ORIENTED_EDGE('',*,*,#3552,.T.);
#4858=ORIENTED_EDGE('',*,*,#3572,.T.);
#4859=ORIENTED_EDGE('',*,*,#3573,.T.);
#4860=ORIENTED_EDGE('',*,*,#3574,.T.);
#4861=ORIENTED_EDGE('',*,*,#3575,.T.);
#4862=ORIENTED_EDGE('',*,*,#3576,.T.);
#4863=ORIENTED_EDGE('',*,*,#3577,.T.);
#4864=ORIENTED_EDGE('',*,*,#3578,.T.);
#4865=ORIENTED_EDGE('',*,*,#3579,.T.);
#4866=ORIENTED_EDGE('',*,*,#3580,.T.);
#4867=ORIENTED_EDGE('',*,*,#3549,.T.);
#4868=ORIENTED_EDGE('',*,*,#3563,.T.);
#4869=ORIENTED_EDGE('',*,*,#3581,.T.);
#4870=ORIENTED_EDGE('',*,*,#3582,.T.);
#4871=ORIENTED_EDGE('',*,*,#3583,.T.);
#4872=ORIENTED_EDGE('',*,*,#3584,.T.);
#4873=ORIENTED_EDGE('',*,*,#3585,.T.);
#4874=ORIENTED_EDGE('',*,*,#3586,.T.);
#4875=ORIENTED_EDGE('',*,*,#3587,.T.);
#4876=ORIENTED_EDGE('',*,*,#3588,.T.);
#4877=ORIENTED_EDGE('',*,*,#3545,.T.);
#4878=ORIENTED_EDGE('',*,*,#3560,.T.);
#4879=ORIENTED_EDGE('',*,*,#3589,.T.);
#4880=ORIENTED_EDGE('',*,*,#3590,.T.);
#4881=ORIENTED_EDGE('',*,*,#3591,.T.);
#4882=ORIENTED_EDGE('',*,*,#3592,.T.);
#4883=ORIENTED_EDGE('',*,*,#3593,.T.);
#4884=ORIENTED_EDGE('',*,*,#3594,.T.);
#4885=ORIENTED_EDGE('',*,*,#3595,.T.);
#4886=ORIENTED_EDGE('',*,*,#3596,.T.);
#4887=ORIENTED_EDGE('',*,*,#3529,.T.);
#4888=ORIENTED_EDGE('',*,*,#3532,.T.);
#4889=ORIENTED_EDGE('',*,*,#3535,.T.);
#4890=ORIENTED_EDGE('',*,*,#3538,.T.);
#4891=ORIENTED_EDGE('',*,*,#3551,.T.);
#4892=ORIENTED_EDGE('',*,*,#3597,.T.);
#4893=ORIENTED_EDGE('',*,*,#3598,.T.);
#4894=ORIENTED_EDGE('',*,*,#3572,.F.);
#4895=ORIENTED_EDGE('',*,*,#3553,.T.);
#4896=ORIENTED_EDGE('',*,*,#3571,.F.);
#4897=ORIENTED_EDGE('',*,*,#3599,.T.);
#4898=ORIENTED_EDGE('',*,*,#3600,.T.);
#4899=ORIENTED_EDGE('',*,*,#3570,.F.);
#4900=ORIENTED_EDGE('',*,*,#3601,.F.);
#4901=ORIENTED_EDGE('',*,*,#3602,.F.);
#4902=ORIENTED_EDGE('',*,*,#3599,.F.);
#4903=ORIENTED_EDGE('',*,*,#3569,.F.);
#4904=ORIENTED_EDGE('',*,*,#3603,.F.);
#4905=ORIENTED_EDGE('',*,*,#3604,.F.);
#4906=ORIENTED_EDGE('',*,*,#3601,.T.);
#4907=ORIENTED_EDGE('',*,*,#3565,.F.);
#4908=ORIENTED_EDGE('',*,*,#3605,.F.);
#4909=ORIENTED_EDGE('',*,*,#3606,.F.);
#4910=ORIENTED_EDGE('',*,*,#3607,.F.);
#4911=ORIENTED_EDGE('',*,*,#3564,.F.);
#4912=ORIENTED_EDGE('',*,*,#3556,.F.);
#4913=ORIENTED_EDGE('',*,*,#3608,.F.);
#4914=ORIENTED_EDGE('',*,*,#3605,.T.);
#4915=ORIENTED_EDGE('',*,*,#3607,.T.);
#4916=ORIENTED_EDGE('',*,*,#3609,.F.);
#4917=ORIENTED_EDGE('',*,*,#3610,.T.);
#4918=ORIENTED_EDGE('',*,*,#3566,.F.);
#4919=ORIENTED_EDGE('',*,*,#3539,.T.);
#4920=ORIENTED_EDGE('',*,*,#3611,.F.);
#4921=ORIENTED_EDGE('',*,*,#3612,.T.);
#4922=ORIENTED_EDGE('',*,*,#3613,.T.);
#4923=ORIENTED_EDGE('',*,*,#3614,.T.);
#4924=ORIENTED_EDGE('',*,*,#3615,.T.);
#4925=ORIENTED_EDGE('',*,*,#3616,.T.);
#4926=ORIENTED_EDGE('',*,*,#3617,.T.);
#4927=ORIENTED_EDGE('',*,*,#3609,.T.);
#4928=ORIENTED_EDGE('',*,*,#3606,.T.);
#4929=ORIENTED_EDGE('',*,*,#3608,.T.);
#4930=ORIENTED_EDGE('',*,*,#3555,.F.);
#4931=ORIENTED_EDGE('',*,*,#3527,.T.);
#4932=ORIENTED_EDGE('',*,*,#3554,.T.);
#4933=ORIENTED_EDGE('',*,*,#3600,.F.);
#4934=ORIENTED_EDGE('',*,*,#3602,.T.);
#4935=ORIENTED_EDGE('',*,*,#3604,.T.);
#4936=ORIENTED_EDGE('',*,*,#3618,.T.);
#4937=ORIENTED_EDGE('',*,*,#3619,.T.);
#4938=ORIENTED_EDGE('',*,*,#3620,.T.);
#4939=ORIENTED_EDGE('',*,*,#3621,.T.);
#4940=ORIENTED_EDGE('',*,*,#3622,.T.);
#4941=ORIENTED_EDGE('',*,*,#3623,.T.);
#4942=ORIENTED_EDGE('',*,*,#3624,.T.);
#4943=ORIENTED_EDGE('',*,*,#3597,.F.);
#4944=ORIENTED_EDGE('',*,*,#3536,.T.);
#4945=ORIENTED_EDGE('',*,*,#3625,.F.);
#4946=ORIENTED_EDGE('',*,*,#3626,.T.);
#4947=ORIENTED_EDGE('',*,*,#3627,.F.);
#4948=ORIENTED_EDGE('',*,*,#3619,.F.);
#4949=ORIENTED_EDGE('',*,*,#3628,.T.);
#4950=ORIENTED_EDGE('',*,*,#3567,.F.);
#4951=ORIENTED_EDGE('',*,*,#3610,.F.);
#4952=ORIENTED_EDGE('',*,*,#3617,.F.);
#4953=ORIENTED_EDGE('',*,*,#3629,.F.);
#4954=ORIENTED_EDGE('',*,*,#3626,.F.);
#4955=ORIENTED_EDGE('',*,*,#3627,.T.);
#4956=ORIENTED_EDGE('',*,*,#3625,.T.);
#4957=ORIENTED_EDGE('',*,*,#3629,.T.);
#4958=ORIENTED_EDGE('',*,*,#3616,.F.);
#4959=ORIENTED_EDGE('',*,*,#3630,.T.);
#4960=ORIENTED_EDGE('',*,*,#3631,.T.);
#4961=ORIENTED_EDGE('',*,*,#3632,.T.);
#4962=ORIENTED_EDGE('',*,*,#3633,.T.);
#4963=ORIENTED_EDGE('',*,*,#3632,.F.);
#4964=ORIENTED_EDGE('',*,*,#3634,.T.);
#4965=ORIENTED_EDGE('',*,*,#3635,.T.);
#4966=ORIENTED_EDGE('',*,*,#3636,.F.);
#4967=ORIENTED_EDGE('',*,*,#3637,.T.);
#4968=ORIENTED_EDGE('',*,*,#3638,.T.);
#4969=ORIENTED_EDGE('',*,*,#3639,.T.);
#4970=ORIENTED_EDGE('',*,*,#3640,.F.);
#4971=ORIENTED_EDGE('',*,*,#3641,.T.);
#4972=ORIENTED_EDGE('',*,*,#3642,.T.);
#4973=ORIENTED_EDGE('',*,*,#3643,.T.);
#4974=ORIENTED_EDGE('',*,*,#3620,.F.);
#4975=ORIENTED_EDGE('',*,*,#3603,.T.);
#4976=ORIENTED_EDGE('',*,*,#3568,.F.);
#4977=ORIENTED_EDGE('',*,*,#3628,.F.);
#4978=ORIENTED_EDGE('',*,*,#3618,.F.);
#4979=ORIENTED_EDGE('',*,*,#3542,.T.);
#4980=ORIENTED_EDGE('',*,*,#3596,.F.);
#4981=ORIENTED_EDGE('',*,*,#3644,.T.);
#4982=ORIENTED_EDGE('',*,*,#3611,.T.);
#4983=ORIENTED_EDGE('',*,*,#3595,.F.);
#4984=ORIENTED_EDGE('',*,*,#3645,.F.);
#4985=ORIENTED_EDGE('',*,*,#3612,.F.);
#4986=ORIENTED_EDGE('',*,*,#3644,.F.);
#4987=ORIENTED_EDGE('',*,*,#3594,.F.);
#4988=ORIENTED_EDGE('',*,*,#3646,.F.);
#4989=ORIENTED_EDGE('',*,*,#3613,.F.);
#4990=ORIENTED_EDGE('',*,*,#3645,.T.);
#4991=ORIENTED_EDGE('',*,*,#3590,.F.);
#4992=ORIENTED_EDGE('',*,*,#3647,.F.);
#4993=ORIENTED_EDGE('',*,*,#3648,.F.);
#4994=ORIENTED_EDGE('',*,*,#3649,.F.);
#4995=ORIENTED_EDGE('',*,*,#3589,.F.);
#4996=ORIENTED_EDGE('',*,*,#3559,.F.);
#4997=ORIENTED_EDGE('',*,*,#3650,.F.);
#4998=ORIENTED_EDGE('',*,*,#3647,.T.);
#4999=ORIENTED_EDGE('',*,*,#3649,.T.);
#5000=ORIENTED_EDGE('',*,*,#3651,.F.);
#5001=ORIENTED_EDGE('',*,*,#3652,.T.);
#5002=ORIENTED_EDGE('',*,*,#3591,.F.);
#5003=ORIENTED_EDGE('',*,*,#3543,.T.);
#5004=ORIENTED_EDGE('',*,*,#3653,.F.);
#5005=ORIENTED_EDGE('',*,*,#3654,.T.);
#5006=ORIENTED_EDGE('',*,*,#3655,.T.);
#5007=ORIENTED_EDGE('',*,*,#3656,.T.);
#5008=ORIENTED_EDGE('',*,*,#3657,.T.);
#5009=ORIENTED_EDGE('',*,*,#3636,.T.);
#5010=ORIENTED_EDGE('',*,*,#3658,.T.);
#5011=ORIENTED_EDGE('',*,*,#3651,.T.);
#5012=ORIENTED_EDGE('',*,*,#3648,.T.);
#5013=ORIENTED_EDGE('',*,*,#3650,.T.);
#5014=ORIENTED_EDGE('',*,*,#3558,.F.);
#5015=ORIENTED_EDGE('',*,*,#3530,.T.);
#5016=ORIENTED_EDGE('',*,*,#3631,.F.);
#5017=ORIENTED_EDGE('',*,*,#3659,.T.);
#5018=ORIENTED_EDGE('',*,*,#3634,.F.);
#5019=ORIENTED_EDGE('',*,*,#3630,.F.);
#5020=ORIENTED_EDGE('',*,*,#3615,.F.);
#5021=ORIENTED_EDGE('',*,*,#3660,.T.);
#5022=ORIENTED_EDGE('',*,*,#3592,.F.);
#5023=ORIENTED_EDGE('',*,*,#3652,.F.);
#5024=ORIENTED_EDGE('',*,*,#3658,.F.);
#5025=ORIENTED_EDGE('',*,*,#3635,.F.);
#5026=ORIENTED_EDGE('',*,*,#3659,.F.);
#5027=ORIENTED_EDGE('',*,*,#3646,.T.);
#5028=ORIENTED_EDGE('',*,*,#3593,.F.);
#5029=ORIENTED_EDGE('',*,*,#3660,.F.);
#5030=ORIENTED_EDGE('',*,*,#3614,.F.);
#5031=ORIENTED_EDGE('',*,*,#3546,.T.);
#5032=ORIENTED_EDGE('',*,*,#3588,.F.);
#5033=ORIENTED_EDGE('',*,*,#3661,.T.);
#5034=ORIENTED_EDGE('',*,*,#3653,.T.);
#5035=ORIENTED_EDGE('',*,*,#3587,.F.);
#5036=ORIENTED_EDGE('',*,*,#3662,.F.);
#5037=ORIENTED_EDGE('',*,*,#3654,.F.);
#5038=ORIENTED_EDGE('',*,*,#3661,.F.);
#5039=ORIENTED_EDGE('',*,*,#3586,.F.);
#5040=ORIENTED_EDGE('',*,*,#3663,.F.);
#5041=ORIENTED_EDGE('',*,*,#3655,.F.);
#5042=ORIENTED_EDGE('',*,*,#3662,.T.);
#5043=ORIENTED_EDGE('',*,*,#3582,.F.);
#5044=ORIENTED_EDGE('',*,*,#3664,.F.);
#5045=ORIENTED_EDGE('',*,*,#3665,.F.);
#5046=ORIENTED_EDGE('',*,*,#3666,.F.);
#5047=ORIENTED_EDGE('',*,*,#3581,.F.);
#5048=ORIENTED_EDGE('',*,*,#3562,.F.);
#5049=ORIENTED_EDGE('',*,*,#3667,.F.);
#5050=ORIENTED_EDGE('',*,*,#3664,.T.);
#5051=ORIENTED_EDGE('',*,*,#3666,.T.);
#5052=ORIENTED_EDGE('',*,*,#3668,.F.);
#5053=ORIENTED_EDGE('',*,*,#3669,.T.);
#5054=ORIENTED_EDGE('',*,*,#3583,.F.);
#5055=ORIENTED_EDGE('',*,*,#3547,.T.);
#5056=ORIENTED_EDGE('',*,*,#3670,.F.);
#5057=ORIENTED_EDGE('',*,*,#3671,.T.);
#5058=ORIENTED_EDGE('',*,*,#3672,.T.);
#5059=ORIENTED_EDGE('',*,*,#3673,.T.);
#5060=ORIENTED_EDGE('',*,*,#3674,.T.);
#5061=ORIENTED_EDGE('',*,*,#3640,.T.);
#5062=ORIENTED_EDGE('',*,*,#3675,.T.);
#5063=ORIENTED_EDGE('',*,*,#3668,.T.);
#5064=ORIENTED_EDGE('',*,*,#3665,.T.);
#5065=ORIENTED_EDGE('',*,*,#3667,.T.);
#5066=ORIENTED_EDGE('',*,*,#3561,.F.);
#5067=ORIENTED_EDGE('',*,*,#3533,.T.);
#5068=ORIENTED_EDGE('',*,*,#3638,.F.);
#5069=ORIENTED_EDGE('',*,*,#3676,.T.);
#5070=ORIENTED_EDGE('',*,*,#3637,.F.);
#5071=ORIENTED_EDGE('',*,*,#3657,.F.);
#5072=ORIENTED_EDGE('',*,*,#3677,.T.);
#5073=ORIENTED_EDGE('',*,*,#3584,.F.);
#5074=ORIENTED_EDGE('',*,*,#3669,.F.);
#5075=ORIENTED_EDGE('',*,*,#3675,.F.);
#5076=ORIENTED_EDGE('',*,*,#3639,.F.);
#5077=ORIENTED_EDGE('',*,*,#3676,.F.);
#5078=ORIENTED_EDGE('',*,*,#3663,.T.);
#5079=ORIENTED_EDGE('',*,*,#3585,.F.);
#5080=ORIENTED_EDGE('',*,*,#3677,.F.);
#5081=ORIENTED_EDGE('',*,*,#3656,.F.);
#5082=ORIENTED_EDGE('',*,*,#3550,.T.);
#5083=ORIENTED_EDGE('',*,*,#3580,.F.);
#5084=ORIENTED_EDGE('',*,*,#3678,.T.);
#5085=ORIENTED_EDGE('',*,*,#3670,.T.);
#5086=ORIENTED_EDGE('',*,*,#3579,.F.);
#5087=ORIENTED_EDGE('',*,*,#3679,.F.);
#5088=ORIENTED_EDGE('',*,*,#3671,.F.);
#5089=ORIENTED_EDGE('',*,*,#3678,.F.);
#5090=ORIENTED_EDGE('',*,*,#3624,.F.);
#5091=ORIENTED_EDGE('',*,*,#3680,.T.);
#5092=ORIENTED_EDGE('',*,*,#3573,.F.);
#5093=ORIENTED_EDGE('',*,*,#3598,.F.);
#5094=ORIENTED_EDGE('',*,*,#3623,.F.);
#5095=ORIENTED_EDGE('',*,*,#3681,.F.);
#5096=ORIENTED_EDGE('',*,*,#3574,.F.);
#5097=ORIENTED_EDGE('',*,*,#3680,.F.);
#5098=ORIENTED_EDGE('',*,*,#3578,.F.);
#5099=ORIENTED_EDGE('',*,*,#3682,.F.);
#5100=ORIENTED_EDGE('',*,*,#3672,.F.);
#5101=ORIENTED_EDGE('',*,*,#3679,.T.);
#5102=ORIENTED_EDGE('',*,*,#3642,.F.);
#5103=ORIENTED_EDGE('',*,*,#3683,.T.);
#5104=ORIENTED_EDGE('',*,*,#3641,.F.);
#5105=ORIENTED_EDGE('',*,*,#3674,.F.);
#5106=ORIENTED_EDGE('',*,*,#3684,.T.);
#5107=ORIENTED_EDGE('',*,*,#3576,.F.);
#5108=ORIENTED_EDGE('',*,*,#3685,.F.);
#5109=ORIENTED_EDGE('',*,*,#3621,.F.);
#5110=ORIENTED_EDGE('',*,*,#3643,.F.);
#5111=ORIENTED_EDGE('',*,*,#3683,.F.);
#5112=ORIENTED_EDGE('',*,*,#3682,.T.);
#5113=ORIENTED_EDGE('',*,*,#3577,.F.);
#5114=ORIENTED_EDGE('',*,*,#3684,.F.);
#5115=ORIENTED_EDGE('',*,*,#3673,.F.);
#5116=ORIENTED_EDGE('',*,*,#3681,.T.);
#5117=ORIENTED_EDGE('',*,*,#3622,.F.);
#5118=ORIENTED_EDGE('',*,*,#3685,.T.);
#5119=ORIENTED_EDGE('',*,*,#3575,.F.);
#5120=ORIENTED_EDGE('',*,*,#3633,.F.);
#5121=ORIENTED_EDGE('',*,*,#3686,.F.);
#5122=ORIENTED_EDGE('',*,*,#3686,.T.);
#5123=ORIENTED_EDGE('',*,*,#3687,.T.);
#5124=ORIENTED_EDGE('',*,*,#3688,.T.);
#5125=ORIENTED_EDGE('',*,*,#3687,.F.);
#5126=ORIENTED_EDGE('',*,*,#3688,.F.);
#5337=CYLINDRICAL_SURFACE('',#6571,0.165);
#5338=CYLINDRICAL_SURFACE('',#6574,0.165);
#5339=CYLINDRICAL_SURFACE('',#6577,0.165);
#5340=CYLINDRICAL_SURFACE('',#6580,0.165);
#5341=CYLINDRICAL_SURFACE('',#6583,1.82);
#5342=CYLINDRICAL_SURFACE('',#6586,1.82);
#5343=CYLINDRICAL_SURFACE('',#6589,1.82);
#5344=CYLINDRICAL_SURFACE('',#6592,1.82);
#5345=CYLINDRICAL_SURFACE('',#6595,3.);
#5346=CYLINDRICAL_SURFACE('',#6598,3.);
#5347=CYLINDRICAL_SURFACE('',#6601,3.);
#5348=CYLINDRICAL_SURFACE('',#6614,3.);
#5349=CYLINDRICAL_SURFACE('',#6616,3.);
#5350=CYLINDRICAL_SURFACE('',#6635,0.32);
#5351=CYLINDRICAL_SURFACE('',#6636,0.7);
#5352=CYLINDRICAL_SURFACE('',#6645,3.);
#5353=CYLINDRICAL_SURFACE('',#6657,0.32);
#5354=CYLINDRICAL_SURFACE('',#6659,3.);
#5355=CYLINDRICAL_SURFACE('',#6671,0.32);
#5356=CYLINDRICAL_SURFACE('',#6673,3.);
#5357=CYLINDRICAL_SURFACE('',#6680,0.32);
#5358=CYLINDRICAL_SURFACE('',#6685,0.5);
#5617=ADVANCED_FACE('',(#903),#5337,.F.);
#5618=ADVANCED_FACE('',(#904),#5338,.F.);
#5619=ADVANCED_FACE('',(#905),#5339,.F.);
#5620=ADVANCED_FACE('',(#906),#5340,.F.);
#5621=ADVANCED_FACE('',(#907),#5341,.F.);
#5622=ADVANCED_FACE('',(#908),#5342,.F.);
#5623=ADVANCED_FACE('',(#909),#5343,.F.);
#5624=ADVANCED_FACE('',(#910),#5344,.F.);
#5625=ADVANCED_FACE('',(#911),#5345,.T.);
#5626=ADVANCED_FACE('',(#912),#5346,.T.);
#5627=ADVANCED_FACE('',(#913),#5347,.T.);
#5628=ADVANCED_FACE('',(#914,#456,#457,#458,#459),#600,.T.);
#5629=ADVANCED_FACE('',(#915),#5348,.T.);
#5630=ADVANCED_FACE('',(#916),#5349,.T.);
#5631=ADVANCED_FACE('',(#917),#601,.F.);
#5632=ADVANCED_FACE('',(#918),#602,.F.);
#5633=ADVANCED_FACE('',(#919),#603,.F.);
#5634=ADVANCED_FACE('',(#920),#604,.F.);
#5635=ADVANCED_FACE('',(#921),#605,.F.);
#5636=ADVANCED_FACE('',(#922,#460),#606,.F.);
#5637=ADVANCED_FACE('',(#923,#461),#607,.F.);
#5638=ADVANCED_FACE('',(#924),#608,.T.);
#5639=ADVANCED_FACE('',(#925),#5350,.F.);
#5640=ADVANCED_FACE('',(#926),#5351,.T.);
#5641=ADVANCED_FACE('',(#927),#609,.F.);
#5642=ADVANCED_FACE('',(#928),#5352,.T.);
#5643=ADVANCED_FACE('',(#929),#610,.F.);
#5644=ADVANCED_FACE('',(#930),#611,.F.);
#5645=ADVANCED_FACE('',(#931),#612,.F.);
#5646=ADVANCED_FACE('',(#932),#613,.F.);
#5647=ADVANCED_FACE('',(#933),#614,.F.);
#5648=ADVANCED_FACE('',(#934,#462),#615,.F.);
#5649=ADVANCED_FACE('',(#935),#616,.T.);
#5650=ADVANCED_FACE('',(#936),#5353,.F.);
#5651=ADVANCED_FACE('',(#937),#617,.F.);
#5652=ADVANCED_FACE('',(#938),#5354,.T.);
#5653=ADVANCED_FACE('',(#939),#618,.F.);
#5654=ADVANCED_FACE('',(#940),#619,.F.);
#5655=ADVANCED_FACE('',(#941),#620,.F.);
#5656=ADVANCED_FACE('',(#942),#621,.F.);
#5657=ADVANCED_FACE('',(#943),#622,.F.);
#5658=ADVANCED_FACE('',(#944,#463),#623,.F.);
#5659=ADVANCED_FACE('',(#945),#624,.T.);
#5660=ADVANCED_FACE('',(#946),#5355,.F.);
#5661=ADVANCED_FACE('',(#947),#625,.F.);
#5662=ADVANCED_FACE('',(#948),#5356,.T.);
#5663=ADVANCED_FACE('',(#949),#626,.F.);
#5664=ADVANCED_FACE('',(#950),#627,.F.);
#5665=ADVANCED_FACE('',(#951),#628,.F.);
#5666=ADVANCED_FACE('',(#952),#629,.F.);
#5667=ADVANCED_FACE('',(#953),#630,.T.);
#5668=ADVANCED_FACE('',(#954),#5357,.F.);
#5669=ADVANCED_FACE('',(#955),#631,.F.);
#5670=ADVANCED_FACE('',(#956),#632,.F.);
#5671=ADVANCED_FACE('',(#957,#464),#633,.F.);
#5672=ADVANCED_FACE('',(#958),#5358,.T.);
#5673=ADVANCED_FACE('',(#959),#634,.F.);
#5730=CLOSED_SHELL('',(#5617,#5618,#5619,#5620,#5621,#5622,#5623,#5624,
#5625,#5626,#5627,#5628,#5629,#5630,#5631,#5632,#5633,#5634,#5635,#5636,
#5637,#5638,#5639,#5640,#5641,#5642,#5643,#5644,#5645,#5646,#5647,#5648,
#5649,#5650,#5651,#5652,#5653,#5654,#5655,#5656,#5657,#5658,#5659,#5660,
#5661,#5662,#5663,#5664,#5665,#5666,#5667,#5668,#5669,#5670,#5671,#5672,
#5673));
#6570=AXIS2_PLACEMENT_3D('',#10305,#8109,#8110);
#6571=AXIS2_PLACEMENT_3D('',#10306,#8111,#8112);
#6572=AXIS2_PLACEMENT_3D('',#10308,#8113,#8114);
#6573=AXIS2_PLACEMENT_3D('',#10311,#8116,#8117);
#6574=AXIS2_PLACEMENT_3D('',#10312,#8118,#8119);
#6575=AXIS2_PLACEMENT_3D('',#10314,#8120,#8121);
#6576=AXIS2_PLACEMENT_3D('',#10317,#8123,#8124);
#6577=AXIS2_PLACEMENT_3D('',#10318,#8125,#8126);
#6578=AXIS2_PLACEMENT_3D('',#10320,#8127,#8128);
#6579=AXIS2_PLACEMENT_3D('',#10323,#8130,#8131);
#6580=AXIS2_PLACEMENT_3D('',#10324,#8132,#8133);
#6581=AXIS2_PLACEMENT_3D('',#10326,#8134,#8135);
#6582=AXIS2_PLACEMENT_3D('',#10329,#8137,#8138);
#6583=AXIS2_PLACEMENT_3D('',#10330,#8139,#8140);
#6584=AXIS2_PLACEMENT_3D('',#10333,#8141,#8142);
#6585=AXIS2_PLACEMENT_3D('',#10337,#8144,#8145);
#6586=AXIS2_PLACEMENT_3D('',#10339,#8147,#8148);
#6587=AXIS2_PLACEMENT_3D('',#10342,#8149,#8150);
#6588=AXIS2_PLACEMENT_3D('',#10346,#8152,#8153);
#6589=AXIS2_PLACEMENT_3D('',#10348,#8155,#8156);
#6590=AXIS2_PLACEMENT_3D('',#10351,#8157,#8158);
#6591=AXIS2_PLACEMENT_3D('',#10355,#8160,#8161);
#6592=AXIS2_PLACEMENT_3D('',#10357,#8163,#8164);
#6593=AXIS2_PLACEMENT_3D('',#10362,#8166,#8167);
#6594=AXIS2_PLACEMENT_3D('',#10365,#8169,#8170);
#6595=AXIS2_PLACEMENT_3D('',#10366,#8171,#8172);
#6596=AXIS2_PLACEMENT_3D('',#10368,#8173,#8174);
#6597=AXIS2_PLACEMENT_3D('',#10371,#8176,#8177);
#6598=AXIS2_PLACEMENT_3D('',#10372,#8178,#8179);
#6599=AXIS2_PLACEMENT_3D('',#10374,#8180,#8181);
#6600=AXIS2_PLACEMENT_3D('',#10377,#8183,#8184);
#6601=AXIS2_PLACEMENT_3D('',#10378,#8185,#8186);
#6602=AXIS2_PLACEMENT_3D('',#10380,#8187,#8188);
#6603=AXIS2_PLACEMENT_3D('',#10383,#8190,#8191);
#6604=AXIS2_PLACEMENT_3D('',#10384,#8192,#8193);
#6605=AXIS2_PLACEMENT_3D('',#10392,#8197,#8198);
#6606=AXIS2_PLACEMENT_3D('',#10399,#8202,#8203);
#6607=AXIS2_PLACEMENT_3D('',#10401,#8204,#8205);
#6608=AXIS2_PLACEMENT_3D('',#10409,#8209,#8210);
#6609=AXIS2_PLACEMENT_3D('',#10416,#8214,#8215);
#6610=AXIS2_PLACEMENT_3D('',#10424,#8219,#8220);
#6611=AXIS2_PLACEMENT_3D('',#10431,#8224,#8225);
#6612=AXIS2_PLACEMENT_3D('',#10439,#8229,#8230);
#6613=AXIS2_PLACEMENT_3D('',#10446,#8234,#8235);
#6614=AXIS2_PLACEMENT_3D('',#10447,#8236,#8237);
#6615=AXIS2_PLACEMENT_3D('',#10449,#8238,#8239);
#6616=AXIS2_PLACEMENT_3D('',#10451,#8241,#8242);
#6617=AXIS2_PLACEMENT_3D('',#10454,#8244,#8245);
#6618=AXIS2_PLACEMENT_3D('',#10455,#8246,#8247);
#6619=AXIS2_PLACEMENT_3D('',#10459,#8250,#8251);
#6620=AXIS2_PLACEMENT_3D('',#10463,#8254,#8255);
#6621=AXIS2_PLACEMENT_3D('',#10469,#8259,#8260);
#6622=AXIS2_PLACEMENT_3D('',#10471,#8262,#8263);
#6623=AXIS2_PLACEMENT_3D('',#10475,#8266,#8267);
#6624=AXIS2_PLACEMENT_3D('',#10477,#8268,#8269);
#6625=AXIS2_PLACEMENT_3D('',#10485,#8273,#8274);
#6626=AXIS2_PLACEMENT_3D('',#10487,#8275,#8276);
#6627=AXIS2_PLACEMENT_3D('',#10488,#8277,#8278);
#6628=AXIS2_PLACEMENT_3D('',#10489,#8279,#8280);
#6629=AXIS2_PLACEMENT_3D('',#10493,#8282,#8283);
#6630=AXIS2_PLACEMENT_3D('',#10495,#8284,#8285);
#6631=AXIS2_PLACEMENT_3D('',#10497,#8286,#8287);
#6632=AXIS2_PLACEMENT_3D('',#10503,#8291,#8292);
#6633=AXIS2_PLACEMENT_3D('',#10506,#8293,#8294);
#6634=AXIS2_PLACEMENT_3D('',#10507,#8295,#8296);
#6635=AXIS2_PLACEMENT_3D('',#10508,#8297,#8298);
#6636=AXIS2_PLACEMENT_3D('',#10512,#8302,#8303);
#6637=AXIS2_PLACEMENT_3D('',#10516,#8305,#8306);
#6638=AXIS2_PLACEMENT_3D('',#10519,#8308,#8309);
#6639=AXIS2_PLACEMENT_3D('',#10521,#8310,#8311);
#6640=AXIS2_PLACEMENT_3D('',#10525,#8313,#8314);
#6641=AXIS2_PLACEMENT_3D('',#10529,#8316,#8317);
#6642=AXIS2_PLACEMENT_3D('',#10533,#8319,#8320);
#6643=AXIS2_PLACEMENT_3D('',#10537,#8322,#8323);
#6644=AXIS2_PLACEMENT_3D('',#10539,#8325,#8326);
#6645=AXIS2_PLACEMENT_3D('',#10540,#8327,#8328);
#6646=AXIS2_PLACEMENT_3D('',#10542,#8330,#8331);
#6647=AXIS2_PLACEMENT_3D('',#10544,#8333,#8334);
#6648=AXIS2_PLACEMENT_3D('',#10546,#8336,#8337);
#6649=AXIS2_PLACEMENT_3D('',#10552,#8341,#8342);
#6650=AXIS2_PLACEMENT_3D('',#10554,#8344,#8345);
#6651=AXIS2_PLACEMENT_3D('',#10558,#8348,#8349);
#6652=AXIS2_PLACEMENT_3D('',#10560,#8350,#8351);
#6653=AXIS2_PLACEMENT_3D('',#10567,#8355,#8356);
#6654=AXIS2_PLACEMENT_3D('',#10568,#8357,#8358);
#6655=AXIS2_PLACEMENT_3D('',#10569,#8359,#8360);
#6656=AXIS2_PLACEMENT_3D('',#10570,#8361,#8362);
#6657=AXIS2_PLACEMENT_3D('',#10571,#8363,#8364);
#6658=AXIS2_PLACEMENT_3D('',#10573,#8366,#8367);
#6659=AXIS2_PLACEMENT_3D('',#10574,#8368,#8369);
#6660=AXIS2_PLACEMENT_3D('',#10576,#8371,#8372);
#6661=AXIS2_PLACEMENT_3D('',#10578,#8374,#8375);
#6662=AXIS2_PLACEMENT_3D('',#10580,#8377,#8378);
#6663=AXIS2_PLACEMENT_3D('',#10586,#8382,#8383);
#6664=AXIS2_PLACEMENT_3D('',#10588,#8385,#8386);
#6665=AXIS2_PLACEMENT_3D('',#10592,#8389,#8390);
#6666=AXIS2_PLACEMENT_3D('',#10594,#8391,#8392);
#6667=AXIS2_PLACEMENT_3D('',#10601,#8396,#8397);
#6668=AXIS2_PLACEMENT_3D('',#10602,#8398,#8399);
#6669=AXIS2_PLACEMENT_3D('',#10603,#8400,#8401);
#6670=AXIS2_PLACEMENT_3D('',#10604,#8402,#8403);
#6671=AXIS2_PLACEMENT_3D('',#10605,#8404,#8405);
#6672=AXIS2_PLACEMENT_3D('',#10607,#8407,#8408);
#6673=AXIS2_PLACEMENT_3D('',#10608,#8409,#8410);
#6674=AXIS2_PLACEMENT_3D('',#10610,#8412,#8413);
#6675=AXIS2_PLACEMENT_3D('',#10612,#8415,#8416);
#6676=AXIS2_PLACEMENT_3D('',#10614,#8418,#8419);
#6677=AXIS2_PLACEMENT_3D('',#10616,#8421,#8422);
#6678=AXIS2_PLACEMENT_3D('',#10618,#8424,#8425);
#6679=AXIS2_PLACEMENT_3D('',#10619,#8426,#8427);
#6680=AXIS2_PLACEMENT_3D('',#10620,#8428,#8429);
#6681=AXIS2_PLACEMENT_3D('',#10623,#8432,#8433);
#6682=AXIS2_PLACEMENT_3D('',#10624,#8434,#8435);
#6683=AXIS2_PLACEMENT_3D('',#10625,#8436,#8437);
#6684=AXIS2_PLACEMENT_3D('',#10627,#8438,#8439);
#6685=AXIS2_PLACEMENT_3D('',#10628,#8440,#8441);
#6686=AXIS2_PLACEMENT_3D('',#10631,#8443,#8444);
#6687=AXIS2_PLACEMENT_3D('',#10632,#8445,#8446);
#8109=DIRECTION('axis',(0.,0.,1.));
#8110=DIRECTION('refdir',(1.,0.,0.));
#8111=DIRECTION('center_axis',(0.,0.,1.));
#8112=DIRECTION('ref_axis',(1.,0.,0.));
#8113=DIRECTION('center_axis',(0.,0.,1.));
#8114=DIRECTION('ref_axis',(1.,0.,0.));
#8115=DIRECTION('',(0.,0.,1.));
#8116=DIRECTION('center_axis',(0.,0.,-1.));
#8117=DIRECTION('ref_axis',(1.,0.,0.));
#8118=DIRECTION('center_axis',(0.,0.,1.));
#8119=DIRECTION('ref_axis',(1.,0.,0.));
#8120=DIRECTION('center_axis',(0.,0.,1.));
#8121=DIRECTION('ref_axis',(1.,0.,0.));
#8122=DIRECTION('',(0.,0.,1.));
#8123=DIRECTION('center_axis',(0.,0.,-1.));
#8124=DIRECTION('ref_axis',(1.,0.,0.));
#8125=DIRECTION('center_axis',(0.,0.,1.));
#8126=DIRECTION('ref_axis',(1.,0.,0.));
#8127=DIRECTION('center_axis',(0.,0.,1.));
#8128=DIRECTION('ref_axis',(1.,0.,0.));
#8129=DIRECTION('',(0.,0.,1.));
#8130=DIRECTION('center_axis',(0.,0.,-1.));
#8131=DIRECTION('ref_axis',(1.,0.,0.));
#8132=DIRECTION('center_axis',(0.,0.,1.));
#8133=DIRECTION('ref_axis',(1.,0.,0.));
#8134=DIRECTION('center_axis',(0.,0.,1.));
#8135=DIRECTION('ref_axis',(1.,0.,0.));
#8136=DIRECTION('',(0.,0.,1.));
#8137=DIRECTION('center_axis',(0.,0.,-1.));
#8138=DIRECTION('ref_axis',(1.,0.,0.));
#8139=DIRECTION('center_axis',(0.,0.,1.));
#8140=DIRECTION('ref_axis',(1.,0.,0.));
#8141=DIRECTION('center_axis',(0.,0.,1.));
#8142=DIRECTION('ref_axis',(1.,0.,0.));
#8143=DIRECTION('',(0.,0.,-1.));
#8144=DIRECTION('center_axis',(0.,0.,-1.));
#8145=DIRECTION('ref_axis',(1.,0.,0.));
#8146=DIRECTION('',(0.,0.,1.));
#8147=DIRECTION('center_axis',(0.,0.,1.));
#8148=DIRECTION('ref_axis',(1.,0.,0.));
#8149=DIRECTION('center_axis',(0.,0.,1.));
#8150=DIRECTION('ref_axis',(1.,0.,0.));
#8151=DIRECTION('',(0.,0.,-1.));
#8152=DIRECTION('center_axis',(0.,0.,-1.));
#8153=DIRECTION('ref_axis',(1.,0.,0.));
#8154=DIRECTION('',(0.,0.,1.));
#8155=DIRECTION('center_axis',(0.,0.,1.));
#8156=DIRECTION('ref_axis',(1.,0.,0.));
#8157=DIRECTION('center_axis',(0.,0.,1.));
#8158=DIRECTION('ref_axis',(1.,0.,0.));
#8159=DIRECTION('',(0.,0.,-1.));
#8160=DIRECTION('center_axis',(0.,0.,-1.));
#8161=DIRECTION('ref_axis',(1.,0.,0.));
#8162=DIRECTION('',(0.,0.,1.));
#8163=DIRECTION('center_axis',(0.,0.,1.));
#8164=DIRECTION('ref_axis',(1.,0.,0.));
#8165=DIRECTION('',(0.,0.,-1.));
#8166=DIRECTION('center_axis',(0.,0.,-1.));
#8167=DIRECTION('ref_axis',(1.,0.,0.));
#8168=DIRECTION('',(0.,0.,1.));
#8169=DIRECTION('center_axis',(0.,0.,1.));
#8170=DIRECTION('ref_axis',(1.,0.,0.));
#8171=DIRECTION('center_axis',(0.,0.,1.));
#8172=DIRECTION('ref_axis',(1.,0.,0.));
#8173=DIRECTION('center_axis',(0.,0.,1.));
#8174=DIRECTION('ref_axis',(1.,0.,0.));
#8175=DIRECTION('',(0.,0.,1.));
#8176=DIRECTION('center_axis',(0.,0.,1.));
#8177=DIRECTION('ref_axis',(1.,0.,0.));
#8178=DIRECTION('center_axis',(0.,0.,1.));
#8179=DIRECTION('ref_axis',(1.,0.,0.));
#8180=DIRECTION('center_axis',(0.,0.,1.));
#8181=DIRECTION('ref_axis',(1.,0.,0.));
#8182=DIRECTION('',(0.,0.,1.));
#8183=DIRECTION('center_axis',(0.,0.,1.));
#8184=DIRECTION('ref_axis',(1.,0.,0.));
#8185=DIRECTION('center_axis',(0.,0.,1.));
#8186=DIRECTION('ref_axis',(1.,0.,0.));
#8187=DIRECTION('center_axis',(0.,0.,1.));
#8188=DIRECTION('ref_axis',(1.,0.,0.));
#8189=DIRECTION('',(0.,0.,1.));
#8190=DIRECTION('center_axis',(0.,0.,1.));
#8191=DIRECTION('ref_axis',(1.,0.,0.));
#8192=DIRECTION('center_axis',(0.,0.,1.));
#8193=DIRECTION('ref_axis',(1.,0.,0.));
#8194=DIRECTION('',(0.,1.,0.));
#8195=DIRECTION('',(1.,0.,0.));
#8196=DIRECTION('',(1.70803542250024E-16,1.,0.));
#8197=DIRECTION('center_axis',(0.,0.,-1.));
#8198=DIRECTION('ref_axis',(1.,0.,0.));
#8199=DIRECTION('',(-3.41607084500048E-16,-1.,0.));
#8200=DIRECTION('',(1.,0.,0.));
#8201=DIRECTION('',(0.,-1.,0.));
#8202=DIRECTION('center_axis',(0.,0.,1.));
#8203=DIRECTION('ref_axis',(1.,0.,0.));
#8204=DIRECTION('center_axis',(0.,0.,1.));
#8205=DIRECTION('ref_axis',(1.,0.,0.));
#8206=DIRECTION('',(-1.,0.,0.));
#8207=DIRECTION('',(0.,1.,0.));
#8208=DIRECTION('',(-1.,0.,0.));
#8209=DIRECTION('center_axis',(0.,0.,-1.));
#8210=DIRECTION('ref_axis',(1.,0.,0.));
#8211=DIRECTION('',(1.,0.,0.));
#8212=DIRECTION('',(0.,1.,0.));
#8213=DIRECTION('',(1.,0.,0.));
#8214=DIRECTION('center_axis',(0.,0.,1.));
#8215=DIRECTION('ref_axis',(1.,0.,0.));
#8216=DIRECTION('',(0.,-1.,0.));
#8217=DIRECTION('',(-1.,0.,0.));
#8218=DIRECTION('',(0.,-1.,0.));
#8219=DIRECTION('center_axis',(0.,0.,-1.));
#8220=DIRECTION('ref_axis',(1.,0.,0.));
#8221=DIRECTION('',(0.,1.,0.));
#8222=DIRECTION('',(-1.,0.,0.));
#8223=DIRECTION('',(0.,1.,0.));
#8224=DIRECTION('center_axis',(0.,0.,1.));
#8225=DIRECTION('ref_axis',(1.,0.,0.));
#8226=DIRECTION('',(1.,-1.11022302462516E-16,0.));
#8227=DIRECTION('',(0.,-1.,0.));
#8228=DIRECTION('',(1.,-1.06752213906265E-16,0.));
#8229=DIRECTION('center_axis',(0.,0.,-1.));
#8230=DIRECTION('ref_axis',(1.,0.,0.));
#8231=DIRECTION('',(-1.,1.28102656687518E-16,0.));
#8232=DIRECTION('',(0.,-1.,0.));
#8233=DIRECTION('',(-1.,5.55111512312578E-17,0.));
#8234=DIRECTION('center_axis',(0.,0.,1.));
#8235=DIRECTION('ref_axis',(1.,0.,0.));
#8236=DIRECTION('center_axis',(0.,0.,1.));
#8237=DIRECTION('ref_axis',(1.,0.,0.));
#8238=DIRECTION('center_axis',(0.,0.,1.));
#8239=DIRECTION('ref_axis',(1.,0.,0.));
#8240=DIRECTION('',(0.,0.,1.));
#8241=DIRECTION('center_axis',(0.,0.,1.));
#8242=DIRECTION('ref_axis',(1.,0.,0.));
#8243=DIRECTION('',(0.,0.,-1.));
#8244=DIRECTION('center_axis',(0.,0.,1.));
#8245=DIRECTION('ref_axis',(1.,0.,0.));
#8246=DIRECTION('center_axis',(1.,0.,0.));
#8247=DIRECTION('ref_axis',(0.,1.,0.));
#8248=DIRECTION('',(0.,0.,1.));
#8249=DIRECTION('',(0.,1.,0.));
#8250=DIRECTION('center_axis',(0.,1.,0.));
#8251=DIRECTION('ref_axis',(-1.,0.,0.));
#8252=DIRECTION('',(0.,0.,1.));
#8253=DIRECTION('',(-1.,0.,0.));
#8254=DIRECTION('center_axis',(0.,1.,0.));
#8255=DIRECTION('ref_axis',(-1.,0.,0.));
#8256=DIRECTION('',(0.,0.,1.));
#8257=DIRECTION('',(-1.,0.,0.));
#8258=DIRECTION('',(0.,0.,-1.));
#8259=DIRECTION('center_axis',(-1.,0.,0.));
#8260=DIRECTION('ref_axis',(0.,-1.,0.));
#8261=DIRECTION('',(0.,-1.,0.));
#8262=DIRECTION('center_axis',(-1.,1.70803542250024E-16,0.));
#8263=DIRECTION('ref_axis',(-1.70803542250024E-16,-1.,0.));
#8264=DIRECTION('',(-1.70803542250024E-16,-1.,0.));
#8265=DIRECTION('',(0.,0.,1.));
#8266=DIRECTION('center_axis',(0.,0.,1.));
#8267=DIRECTION('ref_axis',(1.,0.,0.));
#8268=DIRECTION('center_axis',(0.,0.,1.));
#8269=DIRECTION('ref_axis',(1.,0.,0.));
#8270=DIRECTION('',(1.,-5.55111512312578E-17,0.));
#8271=DIRECTION('',(0.,1.,0.));
#8272=DIRECTION('',(1.,-1.28102656687518E-16,0.));
#8273=DIRECTION('center_axis',(0.,0.,1.));
#8274=DIRECTION('ref_axis',(1.,0.,0.));
#8275=DIRECTION('center_axis',(0.,0.,1.));
#8276=DIRECTION('ref_axis',(1.,0.,0.));
#8277=DIRECTION('center_axis',(0.,0.,1.));
#8278=DIRECTION('ref_axis',(1.,0.,0.));
#8279=DIRECTION('center_axis',(0.,0.,1.));
#8280=DIRECTION('ref_axis',(1.,0.,0.));
#8281=DIRECTION('',(3.41607084500048E-16,1.,0.));
#8282=DIRECTION('center_axis',(0.,0.,1.));
#8283=DIRECTION('ref_axis',(1.,0.,0.));
#8284=DIRECTION('center_axis',(0.,0.,1.));
#8285=DIRECTION('ref_axis',(1.,0.,0.));
#8286=DIRECTION('center_axis',(0.,0.,1.));
#8287=DIRECTION('ref_axis',(1.,0.,0.));
#8288=DIRECTION('',(1.,0.,0.));
#8289=DIRECTION('',(0.,-1.,0.));
#8290=DIRECTION('',(1.,0.,0.));
#8291=DIRECTION('center_axis',(0.,0.,1.));
#8292=DIRECTION('ref_axis',(1.,0.,0.));
#8293=DIRECTION('center_axis',(0.,0.,-1.));
#8294=DIRECTION('ref_axis',(1.,0.,0.));
#8295=DIRECTION('center_axis',(0.,0.,1.));
#8296=DIRECTION('ref_axis',(1.,0.,0.));
#8297=DIRECTION('center_axis',(0.,0.,1.));
#8298=DIRECTION('ref_axis',(1.,0.,0.));
#8299=DIRECTION('',(0.,0.,-1.));
#8300=DIRECTION('',(0.,0.,1.));
#8301=DIRECTION('',(0.,0.,1.));
#8302=DIRECTION('center_axis',(0.,0.,1.));
#8303=DIRECTION('ref_axis',(1.,0.,0.));
#8304=DIRECTION('',(0.,0.,-1.));
#8305=DIRECTION('center_axis',(0.,0.,-1.));
#8306=DIRECTION('ref_axis',(1.,0.,0.));
#8307=DIRECTION('',(0.,0.,-1.));
#8308=DIRECTION('center_axis',(0.,0.,1.));
#8309=DIRECTION('ref_axis',(1.,0.,0.));
#8310=DIRECTION('center_axis',(0.,0.,-1.));
#8311=DIRECTION('ref_axis',(1.,0.,0.));
#8312=DIRECTION('',(0.,0.,1.));
#8313=DIRECTION('center_axis',(0.,0.,1.));
#8314=DIRECTION('ref_axis',(1.,0.,0.));
#8315=DIRECTION('',(0.,0.,-1.));
#8316=DIRECTION('center_axis',(0.,0.,-1.));
#8317=DIRECTION('ref_axis',(1.,0.,0.));
#8318=DIRECTION('',(0.,0.,1.));
#8319=DIRECTION('center_axis',(0.,0.,1.));
#8320=DIRECTION('ref_axis',(1.,0.,0.));
#8321=DIRECTION('',(0.,0.,-1.));
#8322=DIRECTION('center_axis',(0.,0.,-1.));
#8323=DIRECTION('ref_axis',(1.,0.,0.));
#8324=DIRECTION('',(0.,0.,1.));
#8325=DIRECTION('center_axis',(1.,-3.41607084500048E-16,0.));
#8326=DIRECTION('ref_axis',(3.41607084500048E-16,1.,0.));
#8327=DIRECTION('center_axis',(0.,0.,1.));
#8328=DIRECTION('ref_axis',(1.,0.,0.));
#8329=DIRECTION('',(0.,0.,-1.));
#8330=DIRECTION('center_axis',(-5.55111512312578E-17,-1.,0.));
#8331=DIRECTION('ref_axis',(1.,-5.55111512312578E-17,0.));
#8332=DIRECTION('',(0.,0.,1.));
#8333=DIRECTION('center_axis',(1.,0.,0.));
#8334=DIRECTION('ref_axis',(0.,1.,0.));
#8335=DIRECTION('',(0.,0.,1.));
#8336=DIRECTION('center_axis',(1.,0.,0.));
#8337=DIRECTION('ref_axis',(0.,1.,0.));
#8338=DIRECTION('',(0.,0.,1.));
#8339=DIRECTION('',(0.,1.,0.));
#8340=DIRECTION('',(0.,0.,-1.));
#8341=DIRECTION('center_axis',(1.11022302462516E-16,1.,0.));
#8342=DIRECTION('ref_axis',(-1.,1.11022302462516E-16,0.));
#8343=DIRECTION('',(-1.,1.11022302462516E-16,0.));
#8344=DIRECTION('center_axis',(1.06752213906265E-16,1.,0.));
#8345=DIRECTION('ref_axis',(-1.,1.06752213906265E-16,0.));
#8346=DIRECTION('',(-1.,1.06752213906265E-16,0.));
#8347=DIRECTION('',(0.,0.,1.));
#8348=DIRECTION('center_axis',(0.,0.,1.));
#8349=DIRECTION('ref_axis',(1.,0.,0.));
#8350=DIRECTION('center_axis',(0.,0.,1.));
#8351=DIRECTION('ref_axis',(1.,0.,0.));
#8352=DIRECTION('',(0.,-1.,0.));
#8353=DIRECTION('',(1.,0.,0.));
#8354=DIRECTION('',(0.,-1.,0.));
#8355=DIRECTION('center_axis',(0.,0.,1.));
#8356=DIRECTION('ref_axis',(1.,0.,0.));
#8357=DIRECTION('center_axis',(0.,0.,1.));
#8358=DIRECTION('ref_axis',(1.,0.,0.));
#8359=DIRECTION('center_axis',(0.,0.,1.));
#8360=DIRECTION('ref_axis',(1.,0.,0.));
#8361=DIRECTION('center_axis',(0.,0.,1.));
#8362=DIRECTION('ref_axis',(1.,0.,0.));
#8363=DIRECTION('center_axis',(0.,0.,1.));
#8364=DIRECTION('ref_axis',(1.,0.,0.));
#8365=DIRECTION('',(0.,0.,1.));
#8366=DIRECTION('center_axis',(-1.28102656687518E-16,-1.,0.));
#8367=DIRECTION('ref_axis',(1.,-1.28102656687518E-16,0.));
#8368=DIRECTION('center_axis',(0.,0.,1.));
#8369=DIRECTION('ref_axis',(1.,0.,0.));
#8370=DIRECTION('',(0.,0.,-1.));
#8371=DIRECTION('center_axis',(-1.,0.,0.));
#8372=DIRECTION('ref_axis',(0.,-1.,0.));
#8373=DIRECTION('',(0.,0.,1.));
#8374=DIRECTION('center_axis',(0.,-1.,0.));
#8375=DIRECTION('ref_axis',(1.,0.,0.));
#8376=DIRECTION('',(0.,0.,1.));
#8377=DIRECTION('center_axis',(0.,-1.,0.));
#8378=DIRECTION('ref_axis',(1.,0.,0.));
#8379=DIRECTION('',(0.,0.,1.));
#8380=DIRECTION('',(1.,0.,0.));
#8381=DIRECTION('',(0.,0.,-1.));
#8382=DIRECTION('center_axis',(1.,0.,0.));
#8383=DIRECTION('ref_axis',(0.,1.,0.));
#8384=DIRECTION('',(0.,1.,0.));
#8385=DIRECTION('center_axis',(1.,0.,0.));
#8386=DIRECTION('ref_axis',(0.,1.,0.));
#8387=DIRECTION('',(0.,1.,0.));
#8388=DIRECTION('',(0.,0.,1.));
#8389=DIRECTION('center_axis',(0.,0.,1.));
#8390=DIRECTION('ref_axis',(1.,0.,0.));
#8391=DIRECTION('center_axis',(0.,0.,1.));
#8392=DIRECTION('ref_axis',(1.,0.,0.));
#8393=DIRECTION('',(-1.,0.,0.));
#8394=DIRECTION('',(0.,-1.,0.));
#8395=DIRECTION('',(-1.,0.,0.));
#8396=DIRECTION('center_axis',(0.,0.,1.));
#8397=DIRECTION('ref_axis',(1.,0.,0.));
#8398=DIRECTION('center_axis',(0.,0.,1.));
#8399=DIRECTION('ref_axis',(1.,0.,0.));
#8400=DIRECTION('center_axis',(0.,0.,1.));
#8401=DIRECTION('ref_axis',(1.,0.,0.));
#8402=DIRECTION('center_axis',(0.,0.,1.));
#8403=DIRECTION('ref_axis',(1.,0.,0.));
#8404=DIRECTION('center_axis',(0.,0.,1.));
#8405=DIRECTION('ref_axis',(1.,0.,0.));
#8406=DIRECTION('',(0.,0.,1.));
#8407=DIRECTION('center_axis',(-1.,0.,0.));
#8408=DIRECTION('ref_axis',(0.,-1.,0.));
#8409=DIRECTION('center_axis',(0.,0.,1.));
#8410=DIRECTION('ref_axis',(1.,0.,0.));
#8411=DIRECTION('',(0.,0.,-1.));
#8412=DIRECTION('center_axis',(0.,1.,0.));
#8413=DIRECTION('ref_axis',(-1.,0.,0.));
#8414=DIRECTION('',(0.,0.,1.));
#8415=DIRECTION('center_axis',(0.,-1.,0.));
#8416=DIRECTION('ref_axis',(1.,0.,0.));
#8417=DIRECTION('',(0.,0.,1.));
#8418=DIRECTION('center_axis',(-1.,0.,0.));
#8419=DIRECTION('ref_axis',(0.,-1.,0.));
#8420=DIRECTION('',(0.,0.,-1.));
#8421=DIRECTION('center_axis',(-1.,0.,0.));
#8422=DIRECTION('ref_axis',(0.,-1.,0.));
#8423=DIRECTION('',(0.,0.,1.));
#8424=DIRECTION('center_axis',(0.,0.,1.));
#8425=DIRECTION('ref_axis',(1.,0.,0.));
#8426=DIRECTION('center_axis',(0.,0.,1.));
#8427=DIRECTION('ref_axis',(1.,0.,0.));
#8428=DIRECTION('center_axis',(0.,0.,1.));
#8429=DIRECTION('ref_axis',(-1.,1.22464679914735E-16,0.));
#8430=DIRECTION('',(0.,0.,1.));
#8431=DIRECTION('',(0.,0.,1.));
#8432=DIRECTION('center_axis',(0.,1.,0.));
#8433=DIRECTION('ref_axis',(-1.,0.,0.));
#8434=DIRECTION('center_axis',(0.,-1.,0.));
#8435=DIRECTION('ref_axis',(1.,0.,0.));
#8436=DIRECTION('center_axis',(0.,0.,1.));
#8437=DIRECTION('ref_axis',(1.,0.,0.));
#8438=DIRECTION('center_axis',(0.,0.,-1.));
#8439=DIRECTION('ref_axis',(1.,0.,0.));
#8440=DIRECTION('center_axis',(0.,0.,1.));
#8441=DIRECTION('ref_axis',(1.,0.,0.));
#8442=DIRECTION('',(0.,0.,-1.));
#8443=DIRECTION('center_axis',(0.,0.,1.));
#8444=DIRECTION('ref_axis',(1.,0.,0.));
#8445=DIRECTION('center_axis',(0.,0.,1.));
#8446=DIRECTION('ref_axis',(1.,0.,0.));
#10305=CARTESIAN_POINT('',(0.,0.,0.));
#10306=CARTESIAN_POINT('Origin',(2.9698484809835,-1.27279220613579,5.9));
#10307=CARTESIAN_POINT('',(2.8048484809835,-1.27279220613579,6.));
#10308=CARTESIAN_POINT('Origin',(2.9698484809835,-1.27279220613579,6.));
#10309=CARTESIAN_POINT('',(2.8048484809835,-1.27279220613579,6.8));
#10310=CARTESIAN_POINT('',(2.8048484809835,-1.27279220613579,5.9));
#10311=CARTESIAN_POINT('Origin',(2.9698484809835,-1.27279220613579,6.8));
#10312=CARTESIAN_POINT('Origin',(2.9698484809835,1.27279220613579,5.9));
#10313=CARTESIAN_POINT('',(2.8048484809835,1.27279220613579,6.));
#10314=CARTESIAN_POINT('Origin',(2.9698484809835,1.27279220613579,6.));
#10315=CARTESIAN_POINT('',(2.8048484809835,1.27279220613579,6.8));
#10316=CARTESIAN_POINT('',(2.8048484809835,1.27279220613579,5.9));
#10317=CARTESIAN_POINT('Origin',(2.9698484809835,1.27279220613579,6.8));
#10318=CARTESIAN_POINT('Origin',(5.51543289325507,1.27279220613579,5.9));
#10319=CARTESIAN_POINT('',(5.35043289325507,1.27279220613579,6.));
#10320=CARTESIAN_POINT('Origin',(5.51543289325507,1.27279220613579,6.));
#10321=CARTESIAN_POINT('',(5.35043289325507,1.27279220613579,6.8));
#10322=CARTESIAN_POINT('',(5.35043289325507,1.27279220613579,5.9));
#10323=CARTESIAN_POINT('Origin',(5.51543289325507,1.27279220613579,6.8));
#10324=CARTESIAN_POINT('Origin',(5.51543289325507,-1.27279220613579,5.9));
#10325=CARTESIAN_POINT('',(5.35043289325507,-1.27279220613579,6.));
#10326=CARTESIAN_POINT('Origin',(5.51543289325507,-1.27279220613579,6.));
#10327=CARTESIAN_POINT('',(5.35043289325507,-1.27279220613579,6.8));
#10328=CARTESIAN_POINT('',(5.35043289325507,-1.27279220613579,5.9));
#10329=CARTESIAN_POINT('Origin',(5.51543289325507,-1.27279220613579,6.8));
#10330=CARTESIAN_POINT('Origin',(1.24264068711928,-3.,5.9));
#10331=CARTESIAN_POINT('',(3.04549806673909,-2.75079071295314,6.));
#10332=CARTESIAN_POINT('',(1.49184997416615,-1.19714262038019,6.));
#10333=CARTESIAN_POINT('Origin',(1.24264068711928,-3.,6.));
#10334=CARTESIAN_POINT('',(3.04549806673909,-2.75079071295314,6.8));
#10335=CARTESIAN_POINT('',(3.04549806673909,-2.75079071295314,5.9));
#10336=CARTESIAN_POINT('',(1.49184997416615,-1.19714262038019,6.8));
#10337=CARTESIAN_POINT('Origin',(1.24264068711928,-3.,6.8));
#10338=CARTESIAN_POINT('',(1.49184997416615,-1.19714262038019,5.9));
#10339=CARTESIAN_POINT('Origin',(1.24264068711929,3.,5.9));
#10340=CARTESIAN_POINT('',(1.49184997416615,1.19714262038019,6.));
#10341=CARTESIAN_POINT('',(3.04549806673909,2.75079071295314,6.));
#10342=CARTESIAN_POINT('Origin',(1.24264068711929,3.,6.));
#10343=CARTESIAN_POINT('',(1.49184997416615,1.19714262038019,6.8));
#10344=CARTESIAN_POINT('',(1.49184997416615,1.19714262038019,5.9));
#10345=CARTESIAN_POINT('',(3.04549806673909,2.75079071295314,6.8));
#10346=CARTESIAN_POINT('Origin',(1.24264068711929,3.,6.8));
#10347=CARTESIAN_POINT('',(3.04549806673909,2.75079071295314,5.9));
#10348=CARTESIAN_POINT('Origin',(7.24264068711929,3.,5.9));
#10349=CARTESIAN_POINT('',(5.43978330749948,2.75079071295314,6.));
#10350=CARTESIAN_POINT('',(6.99343140007243,1.19714262038019,6.));
#10351=CARTESIAN_POINT('Origin',(7.24264068711929,3.,6.));
#10352=CARTESIAN_POINT('',(5.43978330749948,2.75079071295314,6.8));
#10353=CARTESIAN_POINT('',(5.43978330749948,2.75079071295314,5.9));
#10354=CARTESIAN_POINT('',(6.99343140007243,1.19714262038019,6.8));
#10355=CARTESIAN_POINT('Origin',(7.24264068711929,3.,6.8));
#10356=CARTESIAN_POINT('',(6.99343140007243,1.19714262038019,5.9));
#10357=CARTESIAN_POINT('Origin',(7.24264068711929,-3.,5.9));
#10358=CARTESIAN_POINT('',(6.99343140007242,-1.19714262038019,6.8));
#10359=CARTESIAN_POINT('',(6.99343140007242,-1.19714262038019,6.));
#10360=CARTESIAN_POINT('',(6.99343140007243,-1.19714262038019,5.9));
#10361=CARTESIAN_POINT('',(5.43978330749948,-2.75079071295314,6.8));
#10362=CARTESIAN_POINT('Origin',(7.24264068711929,-3.,6.8));
#10363=CARTESIAN_POINT('',(5.43978330749948,-2.75079071295314,6.));
#10364=CARTESIAN_POINT('',(5.43978330749948,-2.75079071295314,5.9));
#10365=CARTESIAN_POINT('Origin',(7.24264068711929,-3.,6.));
#10366=CARTESIAN_POINT('Origin',(4.24264068711929,0.,6.));
#10367=CARTESIAN_POINT('',(3.81264068711929,-2.96902340846279,6.));
#10368=CARTESIAN_POINT('Origin',(4.24264068711929,0.,6.));
#10369=CARTESIAN_POINT('',(3.81264068711929,-2.96902340846279,6.8));
#10370=CARTESIAN_POINT('',(3.81264068711929,-2.96902340846279,6.));
#10371=CARTESIAN_POINT('Origin',(4.24264068711929,0.,6.8));
#10372=CARTESIAN_POINT('Origin',(4.24264068711929,0.,6.));
#10373=CARTESIAN_POINT('',(1.2736172786565,0.43,6.));
#10374=CARTESIAN_POINT('Origin',(4.24264068711929,0.,6.));
#10375=CARTESIAN_POINT('',(1.2736172786565,0.43,6.8));
#10376=CARTESIAN_POINT('',(1.2736172786565,0.43,6.));
#10377=CARTESIAN_POINT('Origin',(4.24264068711929,0.,6.8));
#10378=CARTESIAN_POINT('Origin',(4.24264068711929,0.,6.));
#10379=CARTESIAN_POINT('',(4.67264068711929,2.96902340846279,6.));
#10380=CARTESIAN_POINT('Origin',(4.24264068711929,0.,6.));
#10381=CARTESIAN_POINT('',(4.67264068711929,2.96902340846279,6.8));
#10382=CARTESIAN_POINT('',(4.67264068711929,2.96902340846279,6.));
#10383=CARTESIAN_POINT('Origin',(4.24264068711929,0.,6.8));
#10384=CARTESIAN_POINT('Origin',(4.24264068711929,0.,6.8));
#10385=CARTESIAN_POINT('',(3.81264068711929,-2.6,6.8));
#10386=CARTESIAN_POINT('',(3.81264068711929,-1.3,6.8));
#10387=CARTESIAN_POINT('',(3.92264068711928,-2.6,6.8));
#10388=CARTESIAN_POINT('',(4.45764068711929,-2.6,6.8));
#10389=CARTESIAN_POINT('',(3.92264068711928,-1.,6.8));
#10390=CARTESIAN_POINT('',(3.92264068711929,-0.5,6.8));
#10391=CARTESIAN_POINT('',(4.56264068711929,-1.,6.8));
#10392=CARTESIAN_POINT('Origin',(4.24264068711929,-1.,6.8));
#10393=CARTESIAN_POINT('',(4.56264068711929,-2.6,6.8));
#10394=CARTESIAN_POINT('',(4.56264068711929,-1.8,6.8));
#10395=CARTESIAN_POINT('',(4.67264068711928,-2.6,6.8));
#10396=CARTESIAN_POINT('',(4.45764068711929,-2.6,6.8));
#10397=CARTESIAN_POINT('',(4.67264068711928,-2.96902340846279,6.8));
#10398=CARTESIAN_POINT('',(4.67264068711929,-1.8,6.8));
#10399=CARTESIAN_POINT('Origin',(4.24264068711929,0.,6.8));
#10400=CARTESIAN_POINT('',(7.21166409558207,-0.43,6.8));
#10401=CARTESIAN_POINT('Origin',(4.24264068711929,0.,6.8));
#10402=CARTESIAN_POINT('',(6.84264068711929,-0.43,6.8));
#10403=CARTESIAN_POINT('',(5.54264068711929,-0.43,6.8));
#10404=CARTESIAN_POINT('',(6.84264068711929,-0.32,6.8));
#10405=CARTESIAN_POINT('',(6.84264068711929,0.215,6.8));
#10406=CARTESIAN_POINT('',(5.24264068711929,-0.32,6.8));
#10407=CARTESIAN_POINT('',(4.74264068711929,-0.32,6.8));
#10408=CARTESIAN_POINT('',(5.24264068711929,0.32,6.8));
#10409=CARTESIAN_POINT('Origin',(5.24264068711929,0.,6.8));
#10410=CARTESIAN_POINT('',(6.84264068711929,0.32,6.8));
#10411=CARTESIAN_POINT('',(6.04264068711929,0.32,6.8));
#10412=CARTESIAN_POINT('',(6.84264068711929,0.43,6.8));
#10413=CARTESIAN_POINT('',(6.84264068711929,0.215,6.8));
#10414=CARTESIAN_POINT('',(7.21166409558207,0.43,6.8));
#10415=CARTESIAN_POINT('',(6.04264068711929,0.43,6.8));
#10416=CARTESIAN_POINT('Origin',(4.24264068711929,0.,6.8));
#10417=CARTESIAN_POINT('',(4.67264068711929,2.6,6.8));
#10418=CARTESIAN_POINT('',(4.67264068711929,1.3,6.8));
#10419=CARTESIAN_POINT('',(4.56264068711929,2.6,6.8));
#10420=CARTESIAN_POINT('',(4.02764068711929,2.6,6.8));
#10421=CARTESIAN_POINT('',(4.56264068711929,1.,6.8));
#10422=CARTESIAN_POINT('',(4.56264068711929,0.5,6.8));
#10423=CARTESIAN_POINT('',(3.92264068711928,1.,6.8));
#10424=CARTESIAN_POINT('Origin',(4.24264068711929,1.,6.8));
#10425=CARTESIAN_POINT('',(3.92264068711929,2.6,6.8));
#10426=CARTESIAN_POINT('',(3.92264068711929,1.8,6.8));
#10427=CARTESIAN_POINT('',(3.81264068711929,2.6,6.8));
#10428=CARTESIAN_POINT('',(4.02764068711929,2.6,6.8));
#10429=CARTESIAN_POINT('',(3.81264068711929,2.96902340846279,6.8));
#10430=CARTESIAN_POINT('',(3.81264068711929,1.8,6.8));
#10431=CARTESIAN_POINT('Origin',(4.24264068711929,0.,6.8));
#10432=CARTESIAN_POINT('',(1.64264068711929,0.43,6.8));
#10433=CARTESIAN_POINT('',(2.94264068711929,0.43,6.8));
#10434=CARTESIAN_POINT('',(1.64264068711929,0.32,6.8));
#10435=CARTESIAN_POINT('',(1.64264068711929,-0.215,6.8));
#10436=CARTESIAN_POINT('',(3.24264068711929,0.32,6.8));
#10437=CARTESIAN_POINT('',(3.74264068711929,0.32,6.8));
#10438=CARTESIAN_POINT('',(3.24264068711929,-0.32,6.8));
#10439=CARTESIAN_POINT('Origin',(3.24264068711929,1.22464679914735E-16,
6.8));
#10440=CARTESIAN_POINT('',(1.64264068711929,-0.32,6.8));
#10441=CARTESIAN_POINT('',(2.44264068711929,-0.32,6.8));
#10442=CARTESIAN_POINT('',(1.64264068711929,-0.43,6.8));
#10443=CARTESIAN_POINT('',(1.64264068711929,-0.215,6.8));
#10444=CARTESIAN_POINT('',(1.2736172786565,-0.43,6.8));
#10445=CARTESIAN_POINT('',(2.44264068711929,-0.43,6.8));
#10446=CARTESIAN_POINT('Origin',(4.24264068711929,0.,6.8));
#10447=CARTESIAN_POINT('Origin',(4.24264068711929,0.,6.));
#10448=CARTESIAN_POINT('',(7.21166409558207,-0.43,6.));
#10449=CARTESIAN_POINT('Origin',(4.24264068711929,0.,6.));
#10450=CARTESIAN_POINT('',(7.21166409558207,-0.43,6.));
#10451=CARTESIAN_POINT('Origin',(4.24264068711929,0.,6.));
#10452=CARTESIAN_POINT('',(4.67264068711928,-2.96902340846279,6.));
#10453=CARTESIAN_POINT('',(4.67264068711928,-2.96902340846279,6.));
#10454=CARTESIAN_POINT('Origin',(4.24264068711929,0.,6.));
#10455=CARTESIAN_POINT('Origin',(4.67264068711928,-3.6,5.9));
#10456=CARTESIAN_POINT('',(4.67264068711928,-2.6,6.));
#10457=CARTESIAN_POINT('',(4.67264068711928,-2.6,5.9));
#10458=CARTESIAN_POINT('',(4.67264068711929,-1.8,6.));
#10459=CARTESIAN_POINT('Origin',(4.67264068711928,-2.6,5.9));
#10460=CARTESIAN_POINT('',(4.56264068711929,-2.6,6.));
#10461=CARTESIAN_POINT('',(4.56264068711929,-2.6,5.9));
#10462=CARTESIAN_POINT('',(4.45764068711929,-2.6,6.));
#10463=CARTESIAN_POINT('Origin',(4.67264068711928,-2.6,5.9));
#10464=CARTESIAN_POINT('',(3.81264068711929,-2.6,6.));
#10465=CARTESIAN_POINT('',(3.81264068711929,-2.6,5.9));
#10466=CARTESIAN_POINT('',(3.92264068711928,-2.6,6.));
#10467=CARTESIAN_POINT('',(4.45764068711929,-2.6,6.));
#10468=CARTESIAN_POINT('',(3.92264068711928,-2.6,5.9));
#10469=CARTESIAN_POINT('Origin',(3.81264068711929,-2.6,5.9));
#10470=CARTESIAN_POINT('',(3.81264068711929,-1.3,6.));
#10471=CARTESIAN_POINT('Origin',(3.92264068711928,-1.,5.9));
#10472=CARTESIAN_POINT('',(3.92264068711928,-1.,6.));
#10473=CARTESIAN_POINT('',(3.92264068711929,-0.5,6.));
#10474=CARTESIAN_POINT('',(3.92264068711928,-1.,5.9));
#10475=CARTESIAN_POINT('Origin',(4.24264068711929,0.,6.));
#10476=CARTESIAN_POINT('',(1.2736172786565,-0.43,6.));
#10477=CARTESIAN_POINT('Origin',(4.24264068711929,0.,6.));
#10478=CARTESIAN_POINT('',(1.64264068711929,-0.43,6.));
#10479=CARTESIAN_POINT('',(2.44264068711929,-0.43,6.));
#10480=CARTESIAN_POINT('',(1.64264068711929,-0.32,6.));
#10481=CARTESIAN_POINT('',(1.64264068711929,-0.215,6.));
#10482=CARTESIAN_POINT('',(3.24264068711929,-0.32,6.));
#10483=CARTESIAN_POINT('',(2.44264068711929,-0.32,6.));
#10484=CARTESIAN_POINT('',(3.54884068711929,-0.0929599913941466,6.));
#10485=CARTESIAN_POINT('Origin',(3.24264068711929,1.22464679914735E-16,
6.));
#10486=CARTESIAN_POINT('',(4.14968069572514,-0.6938,6.));
#10487=CARTESIAN_POINT('Origin',(4.24264068711929,0.,6.));
#10488=CARTESIAN_POINT('Origin',(4.24264068711929,-1.,6.));
#10489=CARTESIAN_POINT('Origin',(4.24264068711929,0.,6.));
#10490=CARTESIAN_POINT('',(4.56264068711929,-1.,6.));
#10491=CARTESIAN_POINT('',(4.56264068711929,-1.8,6.));
#10492=CARTESIAN_POINT('',(4.33560067851344,-0.6938,6.));
#10493=CARTESIAN_POINT('Origin',(4.24264068711929,-1.,6.));
#10494=CARTESIAN_POINT('',(4.93644068711929,-0.0929599913941494,6.));
#10495=CARTESIAN_POINT('Origin',(4.24264068711929,0.,6.));
#10496=CARTESIAN_POINT('',(5.24264068711929,-0.32,6.));
#10497=CARTESIAN_POINT('Origin',(5.24264068711929,0.,6.));
#10498=CARTESIAN_POINT('',(6.84264068711929,-0.32,6.));
#10499=CARTESIAN_POINT('',(4.74264068711929,-0.32,6.));
#10500=CARTESIAN_POINT('',(6.84264068711929,-0.43,6.));
#10501=CARTESIAN_POINT('',(6.84264068711929,0.215,6.));
#10502=CARTESIAN_POINT('',(5.54264068711929,-0.43,6.));
#10503=CARTESIAN_POINT('Origin',(4.24264068711929,-1.,5.9));
#10504=CARTESIAN_POINT('',(4.33560067851343,-0.6938,5.9));
#10505=CARTESIAN_POINT('',(4.14968069572514,-0.6938,5.9));
#10506=CARTESIAN_POINT('Origin',(4.24264068711929,0.,5.9));
#10507=CARTESIAN_POINT('Origin',(4.24264068711929,-1.,5.9));
#10508=CARTESIAN_POINT('Origin',(4.24264068711929,-1.,5.9));
#10509=CARTESIAN_POINT('',(4.33560067851343,-0.6938,5.9));
#10510=CARTESIAN_POINT('',(4.56264068711929,-1.,5.9));
#10511=CARTESIAN_POINT('',(4.14968069572514,-0.6938,5.9));
#10512=CARTESIAN_POINT('Origin',(4.24264068711929,0.,2.95));
#10513=CARTESIAN_POINT('',(3.54884068711929,-0.0929599913941465,5.9));
#10514=CARTESIAN_POINT('',(3.54884068711929,-0.0929599913941465,5.9));
#10515=CARTESIAN_POINT('',(3.54264068711929,-8.57252759403147E-17,5.9));
#10516=CARTESIAN_POINT('Origin',(4.24264068711929,0.,5.9));
#10517=CARTESIAN_POINT('',(3.54264068711929,-8.57252759403147E-17,2.95));
#10518=CARTESIAN_POINT('',(3.54264068711929,-8.57252759403147E-17,2.95));
#10519=CARTESIAN_POINT('Origin',(4.24264068711929,0.,2.95));
#10520=CARTESIAN_POINT('',(3.54884068711929,0.0929599913941467,5.9));
#10521=CARTESIAN_POINT('Origin',(4.24264068711929,0.,5.9));
#10522=CARTESIAN_POINT('',(3.54884068711929,0.0929599913941468,6.));
#10523=CARTESIAN_POINT('',(3.54884068711929,0.0929599913941467,5.9));
#10524=CARTESIAN_POINT('',(4.14968069572514,0.6938,6.));
#10525=CARTESIAN_POINT('Origin',(4.24264068711929,0.,6.));
#10526=CARTESIAN_POINT('',(4.14968069572514,0.6938,5.9));
#10527=CARTESIAN_POINT('',(4.14968069572514,0.6938,5.9));
#10528=CARTESIAN_POINT('',(4.33560067851343,0.6938,5.9));
#10529=CARTESIAN_POINT('Origin',(4.24264068711929,0.,5.9));
#10530=CARTESIAN_POINT('',(4.33560067851344,0.6938,6.));
#10531=CARTESIAN_POINT('',(4.33560067851343,0.6938,5.9));
#10532=CARTESIAN_POINT('',(4.93644068711929,0.0929599913941494,6.));
#10533=CARTESIAN_POINT('Origin',(4.24264068711929,0.,6.));
#10534=CARTESIAN_POINT('',(4.93644068711929,0.0929599913941487,5.9));
#10535=CARTESIAN_POINT('',(4.93644068711929,0.0929599913941487,5.9));
#10536=CARTESIAN_POINT('',(4.93644068711929,-0.0929599913941487,5.9));
#10537=CARTESIAN_POINT('Origin',(4.24264068711929,0.,5.9));
#10538=CARTESIAN_POINT('',(4.93644068711929,-0.0929599913941487,5.9));
#10539=CARTESIAN_POINT('Origin',(4.56264068711929,-3.6,5.9));
#10540=CARTESIAN_POINT('Origin',(4.24264068711929,0.,6.));
#10541=CARTESIAN_POINT('',(1.2736172786565,-0.43,6.));
#10542=CARTESIAN_POINT('Origin',(0.642640687119285,-0.43,5.9));
#10543=CARTESIAN_POINT('',(1.64264068711929,-0.43,5.9));
#10544=CARTESIAN_POINT('Origin',(1.64264068711929,-0.43,5.9));
#10545=CARTESIAN_POINT('',(1.64264068711929,-0.32,5.9));
#10546=CARTESIAN_POINT('Origin',(1.64264068711929,-0.43,5.9));
#10547=CARTESIAN_POINT('',(1.64264068711929,0.43,6.));
#10548=CARTESIAN_POINT('',(1.64264068711929,0.43,5.9));
#10549=CARTESIAN_POINT('',(1.64264068711929,0.32,6.));
#10550=CARTESIAN_POINT('',(1.64264068711929,-0.215,6.));
#10551=CARTESIAN_POINT('',(1.64264068711929,0.32,5.9));
#10552=CARTESIAN_POINT('Origin',(1.64264068711929,0.43,5.9));
#10553=CARTESIAN_POINT('',(2.94264068711929,0.43,6.));
#10554=CARTESIAN_POINT('Origin',(3.24264068711929,0.32,5.9));
#10555=CARTESIAN_POINT('',(3.24264068711929,0.32,6.));
#10556=CARTESIAN_POINT('',(3.74264068711929,0.32,6.));
#10557=CARTESIAN_POINT('',(3.24264068711929,0.32,5.9));
#10558=CARTESIAN_POINT('Origin',(4.24264068711929,0.,6.));
#10559=CARTESIAN_POINT('',(3.81264068711929,2.96902340846279,6.));
#10560=CARTESIAN_POINT('Origin',(4.24264068711929,0.,6.));
#10561=CARTESIAN_POINT('',(3.81264068711929,2.6,6.));
#10562=CARTESIAN_POINT('',(3.81264068711929,1.8,6.));
#10563=CARTESIAN_POINT('',(3.92264068711929,2.6,6.));
#10564=CARTESIAN_POINT('',(4.02764068711929,2.6,6.));
#10565=CARTESIAN_POINT('',(3.92264068711928,1.,6.));
#10566=CARTESIAN_POINT('',(3.92264068711929,1.8,6.));
#10567=CARTESIAN_POINT('Origin',(4.24264068711929,1.,6.));
#10568=CARTESIAN_POINT('Origin',(3.24264068711929,1.22464679914735E-16,
6.));
#10569=CARTESIAN_POINT('Origin',(3.24264068711929,1.11022302462516E-16,
5.9));
#10570=CARTESIAN_POINT('Origin',(3.24264068711929,1.22464679914735E-16,
5.9));
#10571=CARTESIAN_POINT('Origin',(3.24264068711929,1.22464679914735E-16,
5.9));
#10572=CARTESIAN_POINT('',(3.24264068711929,-0.32,5.9));
#10573=CARTESIAN_POINT('Origin',(0.642640687119285,-0.32,5.9));
#10574=CARTESIAN_POINT('Origin',(4.24264068711929,0.,6.));
#10575=CARTESIAN_POINT('',(3.81264068711929,2.96902340846279,6.));
#10576=CARTESIAN_POINT('Origin',(3.81264068711929,3.6,5.9));
#10577=CARTESIAN_POINT('',(3.81264068711929,2.6,5.9));
#10578=CARTESIAN_POINT('Origin',(3.81264068711929,2.6,5.9));
#10579=CARTESIAN_POINT('',(3.92264068711928,2.6,5.9));
#10580=CARTESIAN_POINT('Origin',(3.81264068711929,2.6,5.9));
#10581=CARTESIAN_POINT('',(4.67264068711929,2.6,6.));
#10582=CARTESIAN_POINT('',(4.67264068711929,2.6,5.9));
#10583=CARTESIAN_POINT('',(4.56264068711929,2.6,6.));
#10584=CARTESIAN_POINT('',(4.02764068711929,2.6,6.));
#10585=CARTESIAN_POINT('',(4.56264068711929,2.6,5.9));
#10586=CARTESIAN_POINT('Origin',(4.67264068711929,2.6,5.9));
#10587=CARTESIAN_POINT('',(4.67264068711929,1.3,6.));
#10588=CARTESIAN_POINT('Origin',(4.56264068711929,1.,5.9));
#10589=CARTESIAN_POINT('',(4.56264068711929,1.,6.));
#10590=CARTESIAN_POINT('',(4.56264068711929,0.5,6.));
#10591=CARTESIAN_POINT('',(4.56264068711929,1.,5.9));
#10592=CARTESIAN_POINT('Origin',(4.24264068711929,0.,6.));
#10593=CARTESIAN_POINT('',(7.21166409558207,0.43,6.));
#10594=CARTESIAN_POINT('Origin',(4.24264068711929,0.,6.));
#10595=CARTESIAN_POINT('',(6.84264068711929,0.43,6.));
#10596=CARTESIAN_POINT('',(6.04264068711929,0.43,6.));
#10597=CARTESIAN_POINT('',(6.84264068711929,0.32,6.));
#10598=CARTESIAN_POINT('',(6.84264068711929,0.215,6.));
#10599=CARTESIAN_POINT('',(5.24264068711929,0.32,6.));
#10600=CARTESIAN_POINT('',(6.04264068711929,0.32,6.));
#10601=CARTESIAN_POINT('Origin',(5.24264068711929,0.,6.));
#10602=CARTESIAN_POINT('Origin',(4.24264068711929,1.,6.));
#10603=CARTESIAN_POINT('Origin',(4.24264068711929,1.,5.9));
#10604=CARTESIAN_POINT('Origin',(4.24264068711929,1.,5.9));
#10605=CARTESIAN_POINT('Origin',(4.24264068711929,1.,5.9));
#10606=CARTESIAN_POINT('',(3.92264068711928,1.,5.9));
#10607=CARTESIAN_POINT('Origin',(3.92264068711928,3.6,5.9));
#10608=CARTESIAN_POINT('Origin',(4.24264068711929,0.,6.));
#10609=CARTESIAN_POINT('',(7.21166409558207,0.43,6.));
#10610=CARTESIAN_POINT('Origin',(7.84264068711929,0.43,5.9));
#10611=CARTESIAN_POINT('',(6.84264068711929,0.43,5.9));
#10612=CARTESIAN_POINT('Origin',(6.84264068711929,-0.43,5.9));
#10613=CARTESIAN_POINT('',(6.84264068711929,-0.43,5.9));
#10614=CARTESIAN_POINT('Origin',(6.84264068711929,0.43,5.9));
#10615=CARTESIAN_POINT('',(6.84264068711929,-0.32,5.9));
#10616=CARTESIAN_POINT('Origin',(6.84264068711929,0.43,5.9));
#10617=CARTESIAN_POINT('',(6.84264068711929,0.32,5.9));
#10618=CARTESIAN_POINT('Origin',(5.24264068711929,0.,5.9));
#10619=CARTESIAN_POINT('Origin',(5.24264068711929,0.,5.9));
#10620=CARTESIAN_POINT('Origin',(5.24264068711929,0.,5.9));
#10621=CARTESIAN_POINT('',(5.24264068711929,0.32,5.9));
#10622=CARTESIAN_POINT('',(5.24264068711929,-0.32,5.9));
#10623=CARTESIAN_POINT('Origin',(7.84264068711929,0.32,5.9));
#10624=CARTESIAN_POINT('Origin',(5.24264068711929,-0.32,5.9));
#10625=CARTESIAN_POINT('Origin',(4.24264068711929,0.,2.95));
#10626=CARTESIAN_POINT('',(3.74264068711929,6.12323399573677E-17,2.95));
#10627=CARTESIAN_POINT('Origin',(4.24264068711929,0.,2.95));
#10628=CARTESIAN_POINT('Origin',(4.24264068711929,0.,1.));
#10629=CARTESIAN_POINT('',(3.74264068711929,-6.12323399573677E-17,1.));
#10630=CARTESIAN_POINT('',(3.74264068711929,-6.12323399573677E-17,1.));
#10631=CARTESIAN_POINT('Origin',(4.24264068711929,0.,1.));
#10632=CARTESIAN_POINT('Origin',(4.24264068711929,0.,1.));
#10922=UNCERTAINTY_MEASURE_WITH_UNIT(LENGTH_MEASURE(0.001),#10958,
'DISTANCE_ACCURACY_VALUE',
'Maximum model space distance between geometric entities at asserted c
onnectivities');
#10926=UNCERTAINTY_MEASURE_WITH_UNIT(LENGTH_MEASURE(0.001),#10958,
'DISTANCE_ACCURACY_VALUE',
'Maximum model space distance between geometric entities at asserted c
onnectivities');
#10953=(
GEOMETRIC_REPRESENTATION_CONTEXT(3)
GLOBAL_UNCERTAINTY_ASSIGNED_CONTEXT((#10922))
GLOBAL_UNIT_ASSIGNED_CONTEXT((#10958,#10960,#10961))
REPRESENTATION_CONTEXT('','3D')
);
#10957=(
GEOMETRIC_REPRESENTATION_CONTEXT(3)
GLOBAL_UNCERTAINTY_ASSIGNED_CONTEXT((#10926))
GLOBAL_UNIT_ASSIGNED_CONTEXT((#10958,#10960,#10961))
REPRESENTATION_CONTEXT('','3D')
);
#10958=(
LENGTH_UNIT()
NAMED_UNIT(*)
SI_UNIT(.CENTI.,.METRE.)
);
#10960=(
NAMED_UNIT(*)
PLANE_ANGLE_UNIT()
SI_UNIT($,.RADIAN.)
);
#10961=(
NAMED_UNIT(*)
SI_UNIT($,.STERADIAN.)
SOLID_ANGLE_UNIT()
);
#10988=SHAPE_DEFINITION_REPRESENTATION(#11043,#11090);
#11043=PRODUCT_DEFINITION_SHAPE('',$,#11121);
#11090=SHAPE_REPRESENTATION('',(#6570),#10953);
#11094=PRODUCT_DEFINITION_CONTEXT('part definition',#11186,'design');
#11121=PRODUCT_DEFINITION('Output wheel and spindle',
'Output wheel and spindle',#11151,#11094);
#11151=PRODUCT_DEFINITION_FORMATION('',$,#11214);
#11186=APPLICATION_CONTEXT(
'Core Data for Automotive Mechanical Design Process');
#11187=PRODUCT_CONTEXT('part definition',#11186,'mechanical');
#11214=PRODUCT('Output wheel and spindle','Output wheel and spindle',
'Output wheel and spindle',(#11187));
#11274=COLOUR_RGB('Sky Blue',0.24,0.69,0.87);
#11275=FILL_AREA_STYLE_COLOUR('',#11274);
#11276=FILL_AREA_STYLE('',(#11275));
#11277=SURFACE_STYLE_FILL_AREA(#11276);
#11278=SURFACE_SIDE_STYLE('',(#11277));
#11279=SURFACE_STYLE_USAGE(.BOTH.,#11278);
#11280=PRESENTATION_STYLE_ASSIGNMENT((#11279));
ENDSEC;
END-ISO-10303-21;
